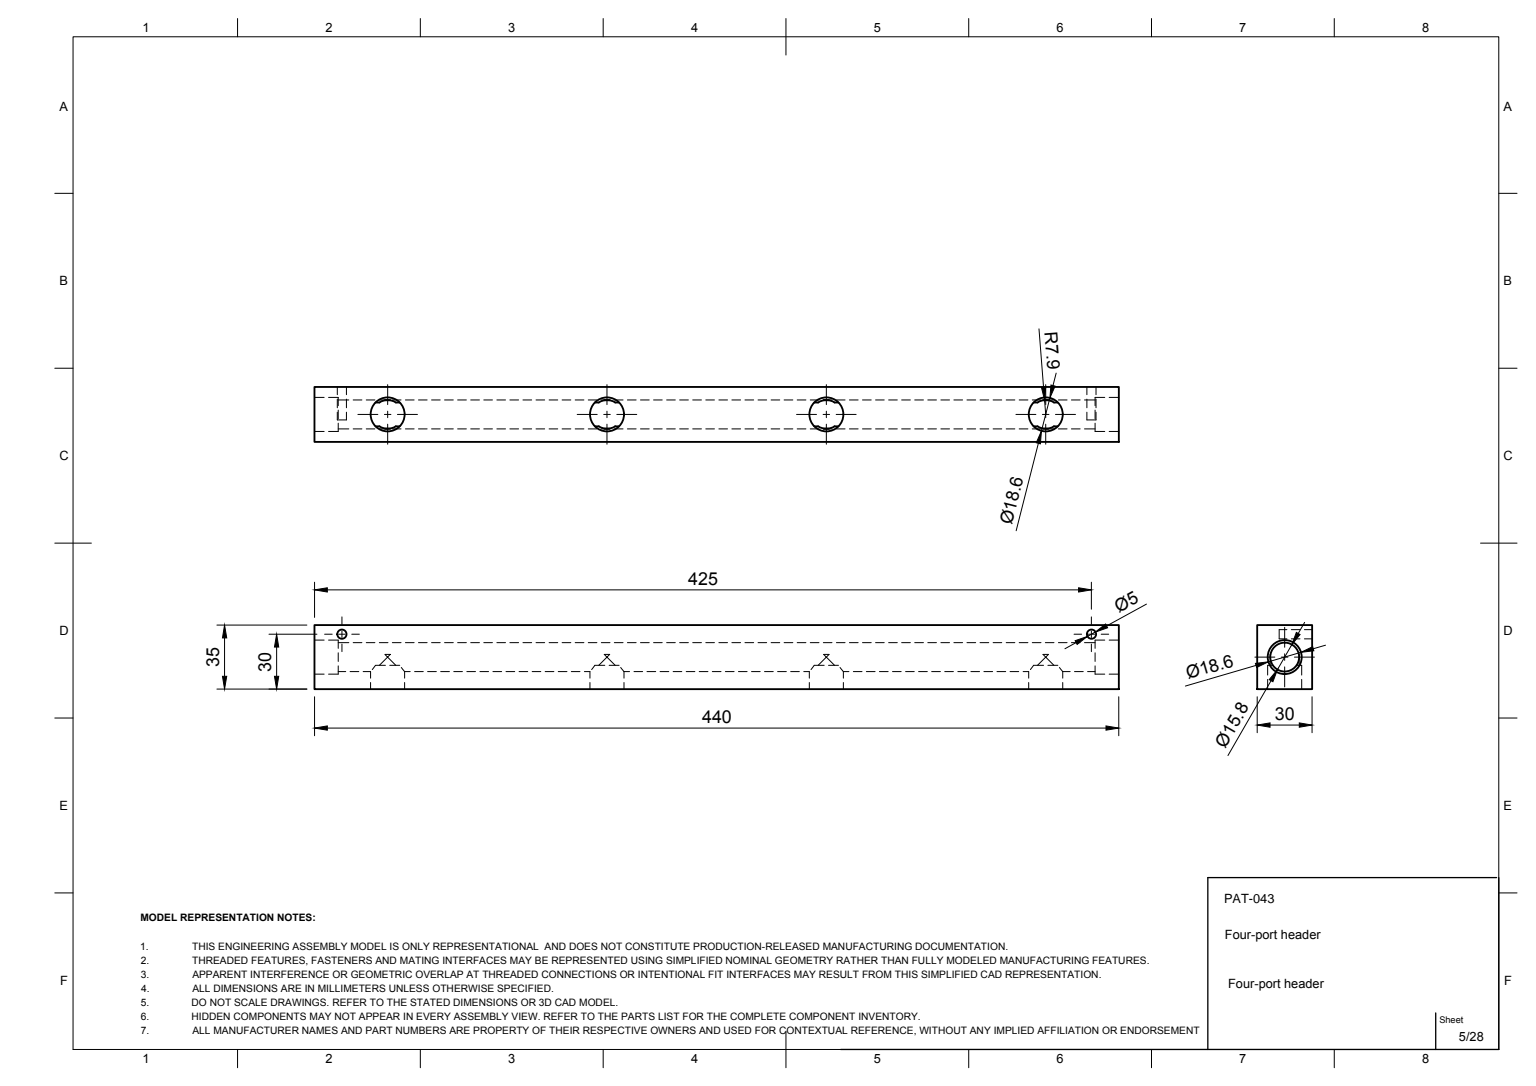
ISO-10303-21;
HEADER;
/* Generated by software containing ST-Developer
 * from STEP Tools, Inc. (www.steptools.com) 
 */

FILE_DESCRIPTION(
/* description */ ('Four-valve pipe header'),
/* implementation_level */ '2;1');

FILE_NAME(
/* name */ 'Four-port header.step',
/* time_stamp */ '2026-10-29T16:56:19-07:00',
/* author */ (''),
/* organization */ (''),
/* preprocessor_version */ 'ST-DEVELOPER v20.2',
/* originating_system */ 'Autodesk Translation Framework v15.17.0.0',
/* authorisation */ '');

FILE_SCHEMA (('AUTOMOTIVE_DESIGN { 1 0 10303 214 3 1 1 }'));
ENDSEC;

DATA;
#10=MECHANICAL_DESIGN_GEOMETRIC_PRESENTATION_REPRESENTATION('',(#333),#10119);
#281=SHAPE_REPRESENTATION_RELATIONSHIP('SRR','None',#10242,#307);
#307=ADVANCED_BREP_SHAPE_REPRESENTATION('',(#359),#10091);
#333=STYLED_ITEM('',(#10484),#359);
#359=MANIFOLD_SOLID_BREP('Body1',#5579);
#382=B_SPLINE_CURVE_WITH_KNOTS('',3,(#8408,#8409,#8410,#8411,#8412,#8413,
#8414,#8415),.UNSPECIFIED.,.F.,.F.,(4,2,2,4),(3.10041913490528,3.25801314591541,
3.57457123454079,3.89112932316618),.UNSPECIFIED.);
#383=B_SPLINE_CURVE_WITH_KNOTS('',3,(#8417,#8418,#8419,#8420,#8421,#8422,
#8423,#8424),.UNSPECIFIED.,.F.,.F.,(4,2,2,4),(3.89112932316618,4.20768741179156,
4.52424550041694,4.68183951142707),.UNSPECIFIED.);
#384=B_SPLINE_CURVE_WITH_KNOTS('',3,(#8439,#8440,#8441,#8442,#8443,#8444,
#8445,#8446,#8447,#8448,#8449,#8450,#8451,#8452),.UNSPECIFIED.,.F.,.F.,
(4,2,2,2,2,2,4),(0.506332919461168,0.663926930471297,0.980485019096678,
1.29704310772206,1.61360119634744,1.93015928497282,2.08775329598295),
 .UNSPECIFIED.);
#385=B_SPLINE_CURVE_WITH_KNOTS('',3,(#8463,#8464,#8465,#8466,#8467,#8468,
#8469,#8470),.UNSPECIFIED.,.F.,.F.,(4,2,2,4),(3.10041913490528,3.25801314591541,
3.5745712345408,3.89112932316618),.UNSPECIFIED.);
#386=B_SPLINE_CURVE_WITH_KNOTS('',3,(#8472,#8473,#8474,#8475,#8476,#8477,
#8478,#8479),.UNSPECIFIED.,.F.,.F.,(4,2,2,4),(3.89112932316618,4.20768741179156,
4.52424550041694,4.68183951142707),.UNSPECIFIED.);
#387=B_SPLINE_CURVE_WITH_KNOTS('',3,(#8494,#8495,#8496,#8497,#8498,#8499,
#8500,#8501,#8502,#8503,#8504,#8505,#8506,#8507),.UNSPECIFIED.,.F.,.F.,
(4,2,2,2,2,2,4),(0.506332919461167,0.663926930471296,0.980485019096678,
1.29704310772206,1.61360119634744,1.93015928497282,2.08775329598295),
 .UNSPECIFIED.);
#388=B_SPLINE_CURVE_WITH_KNOTS('',3,(#8518,#8519,#8520,#8521,#8522,#8523,
#8524,#8525),.UNSPECIFIED.,.F.,.F.,(4,2,2,4),(3.10041913490528,3.25801314591541,
3.5745712345408,3.89112932316618),.UNSPECIFIED.);
#389=B_SPLINE_CURVE_WITH_KNOTS('',3,(#8527,#8528,#8529,#8530,#8531,#8532,
#8533,#8534),.UNSPECIFIED.,.F.,.F.,(4,2,2,4),(3.89112932316618,4.20768741179156,
4.52424550041694,4.68183951142707),.UNSPECIFIED.);
#390=B_SPLINE_CURVE_WITH_KNOTS('',3,(#8549,#8550,#8551,#8552,#8553,#8554,
#8555,#8556,#8557,#8558,#8559,#8560,#8561,#8562),.UNSPECIFIED.,.F.,.F.,
(4,2,2,2,2,2,4),(0.506332919461169,0.663926930471296,0.980485019096678,
1.29704310772206,1.61360119634744,1.93015928497282,2.08775329598295),
 .UNSPECIFIED.);
#391=B_SPLINE_CURVE_WITH_KNOTS('',3,(#8570,#8571,#8572,#8573,#8574,#8575,
#8576,#8577),.UNSPECIFIED.,.F.,.F.,(4,2,2,4),(3.10041913490528,3.25801314591541,
3.5745712345408,3.89112932316618),.UNSPECIFIED.);
#392=B_SPLINE_CURVE_WITH_KNOTS('',3,(#8579,#8580,#8581,#8582,#8583,#8584,
#8585,#8586),.UNSPECIFIED.,.F.,.F.,(4,2,2,4),(3.89112932316618,4.20768741179156,
4.52424550041694,4.68183951142707),.UNSPECIFIED.);
#393=B_SPLINE_CURVE_WITH_KNOTS('',3,(#8591,#8592,#8593,#8594,#8595,#8596,
#8597,#8598,#8599,#8600,#8601,#8602,#8603,#8604),.UNSPECIFIED.,.F.,.F.,
(4,2,2,2,2,2,4),(0.506332919461165,0.663926930471296,0.980485019096678,
1.29704310772206,1.61360119634744,1.93015928497282,2.08775329598295),
 .UNSPECIFIED.);
#394=ELLIPSE('',#5919,1.11722871427474,0.789999999999999);
#395=ELLIPSE('',#5920,1.11722871427474,0.789999999999999);
#396=ELLIPSE('',#5922,1.11722871427474,0.789999999999999);
#397=ELLIPSE('',#5924,1.11722871427474,0.789999999999999);
#398=ELLIPSE('',#5926,1.11722871427474,0.789999999999999);
#399=ELLIPSE('',#5927,1.11722871427474,0.789999999999999);
#400=ELLIPSE('',#5930,1.11722871427474,0.789999999999999);
#401=ELLIPSE('',#5931,1.11722871427474,0.789999999999999);
#402=ELLIPSE('',#5935,1.11722871427474,0.79);
#403=ELLIPSE('',#5936,1.11722871427474,0.79);
#404=ELLIPSE('',#5937,1.11722871427475,0.79);
#405=ELLIPSE('',#5938,1.11722871427474,0.79);
#406=ELLIPSE('',#5939,1.11722871427475,0.79);
#407=ELLIPSE('',#5940,1.11722871427475,0.79);
#408=ELLIPSE('',#5941,1.11722871427474,0.789999999999999);
#409=ELLIPSE('',#5942,1.11722871427474,0.789999999999999);
#410=ELLIPSE('',#5943,1.11722871427474,0.789999999999999);
#411=ELLIPSE('',#5944,1.11722871427474,0.789999999999999);
#412=ELLIPSE('',#5945,1.11722871427474,0.789999999999999);
#413=ELLIPSE('',#5946,1.11722871427474,0.789999999999999);
#414=ELLIPSE('',#5947,1.11722871427474,0.789999999999999);
#415=ELLIPSE('',#5948,1.11722871427474,0.789999999999999);
#416=ELLIPSE('',#5949,1.11722871427474,0.789999999999999);
#417=ELLIPSE('',#5950,1.11722871427474,0.789999999999999);
#418=ELLIPSE('',#5951,1.11722871427474,0.789999999999999);
#419=ELLIPSE('',#5952,1.11722871427474,0.789999999999999);
#420=ELLIPSE('',#5953,1.11722871427474,0.789999999999999);
#421=ELLIPSE('',#5954,1.11722871427474,0.789999999999999);
#422=ELLIPSE('',#5955,1.11722871427474,0.789999999999999);
#423=ELLIPSE('',#5956,1.11722871427474,0.789999999999999);
#424=ELLIPSE('',#5957,1.11722871427474,0.79);
#425=ELLIPSE('',#5958,1.11722871427475,0.79);
#426=FACE_BOUND('',#1085,.T.);
#427=FACE_BOUND('',#1088,.T.);
#428=FACE_BOUND('',#1128,.T.);
#429=FACE_BOUND('',#1130,.T.);
#430=FACE_BOUND('',#1131,.T.);
#431=FACE_BOUND('',#1132,.T.);
#432=FACE_BOUND('',#1133,.T.);
#433=FACE_BOUND('',#1135,.T.);
#434=FACE_BOUND('',#1138,.T.);
#435=FACE_BOUND('',#1139,.T.);
#535=PLANE('',#5901);
#536=PLANE('',#5905);
#537=PLANE('',#5909);
#538=PLANE('',#5914);
#539=PLANE('',#5916);
#540=PLANE('',#5933);
#541=PLANE('',#5959);
#542=PLANE('',#5964);
#543=PLANE('',#5965);
#544=PLANE('',#5974);
#545=PLANE('',#5975);
#546=PLANE('',#5980);
#547=PLANE('',#5981);
#548=PLANE('',#5990);
#549=PLANE('',#5991);
#550=PLANE('',#5996);
#551=PLANE('',#5997);
#552=PLANE('',#6006);
#553=PLANE('',#6007);
#554=PLANE('',#6012);
#555=PLANE('',#6013);
#556=PLANE('',#6014);
#557=PLANE('',#6015);
#558=PLANE('',#6016);
#559=PLANE('',#6017);
#560=PLANE('',#6018);
#747=FACE_OUTER_BOUND('',#1079,.T.);
#748=FACE_OUTER_BOUND('',#1080,.T.);
#749=FACE_OUTER_BOUND('',#1081,.T.);
#750=FACE_OUTER_BOUND('',#1082,.T.);
#751=FACE_OUTER_BOUND('',#1083,.T.);
#752=FACE_OUTER_BOUND('',#1084,.T.);
#753=FACE_OUTER_BOUND('',#1086,.T.);
#754=FACE_OUTER_BOUND('',#1087,.T.);
#755=FACE_OUTER_BOUND('',#1089,.T.);
#756=FACE_OUTER_BOUND('',#1090,.T.);
#757=FACE_OUTER_BOUND('',#1091,.T.);
#758=FACE_OUTER_BOUND('',#1092,.T.);
#759=FACE_OUTER_BOUND('',#1093,.T.);
#760=FACE_OUTER_BOUND('',#1094,.T.);
#761=FACE_OUTER_BOUND('',#1095,.T.);
#762=FACE_OUTER_BOUND('',#1096,.T.);
#763=FACE_OUTER_BOUND('',#1097,.T.);
#764=FACE_OUTER_BOUND('',#1098,.T.);
#765=FACE_OUTER_BOUND('',#1099,.T.);
#766=FACE_OUTER_BOUND('',#1100,.T.);
#767=FACE_OUTER_BOUND('',#1101,.T.);
#768=FACE_OUTER_BOUND('',#1102,.T.);
#769=FACE_OUTER_BOUND('',#1103,.T.);
#770=FACE_OUTER_BOUND('',#1104,.T.);
#771=FACE_OUTER_BOUND('',#1105,.T.);
#772=FACE_OUTER_BOUND('',#1106,.T.);
#773=FACE_OUTER_BOUND('',#1107,.T.);
#774=FACE_OUTER_BOUND('',#1108,.T.);
#775=FACE_OUTER_BOUND('',#1109,.T.);
#776=FACE_OUTER_BOUND('',#1110,.T.);
#777=FACE_OUTER_BOUND('',#1111,.T.);
#778=FACE_OUTER_BOUND('',#1112,.T.);
#779=FACE_OUTER_BOUND('',#1113,.T.);
#780=FACE_OUTER_BOUND('',#1114,.T.);
#781=FACE_OUTER_BOUND('',#1115,.T.);
#782=FACE_OUTER_BOUND('',#1116,.T.);
#783=FACE_OUTER_BOUND('',#1117,.T.);
#784=FACE_OUTER_BOUND('',#1118,.T.);
#785=FACE_OUTER_BOUND('',#1119,.T.);
#786=FACE_OUTER_BOUND('',#1120,.T.);
#787=FACE_OUTER_BOUND('',#1121,.T.);
#788=FACE_OUTER_BOUND('',#1122,.T.);
#789=FACE_OUTER_BOUND('',#1123,.T.);
#790=FACE_OUTER_BOUND('',#1124,.T.);
#791=FACE_OUTER_BOUND('',#1125,.T.);
#792=FACE_OUTER_BOUND('',#1126,.T.);
#793=FACE_OUTER_BOUND('',#1127,.T.);
#794=FACE_OUTER_BOUND('',#1129,.T.);
#795=FACE_OUTER_BOUND('',#1134,.T.);
#796=FACE_OUTER_BOUND('',#1136,.T.);
#797=FACE_OUTER_BOUND('',#1137,.T.);
#1079=EDGE_LOOP('',(#3741,#3742,#3743,#3744));
#1080=EDGE_LOOP('',(#3745));
#1081=EDGE_LOOP('',(#3746,#3747,#3748,#3749));
#1082=EDGE_LOOP('',(#3750));
#1083=EDGE_LOOP('',(#3751,#3752,#3753,#3754));
#1084=EDGE_LOOP('',(#3755));
#1085=EDGE_LOOP('',(#3756));
#1086=EDGE_LOOP('',(#3757,#3758,#3759,#3760));
#1087=EDGE_LOOP('',(#3761));
#1088=EDGE_LOOP('',(#3762));
#1089=EDGE_LOOP('',(#3763,#3764));
#1090=EDGE_LOOP('',(#3765,#3766,#3767));
#1091=EDGE_LOOP('',(#3768,#3769,#3770));
#1092=EDGE_LOOP('',(#3771,#3772,#3773));
#1093=EDGE_LOOP('',(#3774,#3775,#3776));
#1094=EDGE_LOOP('',(#3777,#3778));
#1095=EDGE_LOOP('',(#3779,#3780,#3781,#3782,#3783,#3784,#3785,#3786,#3787,
#3788,#3789,#3790,#3791,#3792,#3793,#3794,#3795,#3796,#3797,#3798,#3799,
#3800,#3801,#3802,#3803,#3804,#3805,#3806,#3807,#3808,#3809,#3810,#3811,
#3812,#3813,#3814,#3815,#3816,#3817,#3818,#3819,#3820,#3821,#3822,#3823,
#3824,#3825,#3826,#3827,#3828,#3829,#3830,#3831,#3832,#3833,#3834,#3835,
#3836,#3837,#3838,#3839,#3840,#3841,#3842,#3843,#3844,#3845,#3846,#3847,
#3848,#3849,#3850,#3851,#3852,#3853,#3854,#3855,#3856,#3857,#3858));
#1096=EDGE_LOOP('',(#3859,#3860,#3861,#3862));
#1097=EDGE_LOOP('',(#3863,#3864,#3865,#3866,#3867,#3868,#3869,#3870));
#1098=EDGE_LOOP('',(#3871,#3872,#3873,#3874));
#1099=EDGE_LOOP('',(#3875,#3876));
#1100=EDGE_LOOP('',(#3877,#3878,#3879));
#1101=EDGE_LOOP('',(#3880,#3881,#3882));
#1102=EDGE_LOOP('',(#3883,#3884,#3885));
#1103=EDGE_LOOP('',(#3886,#3887,#3888));
#1104=EDGE_LOOP('',(#3889,#3890));
#1105=EDGE_LOOP('',(#3891,#3892,#3893,#3894));
#1106=EDGE_LOOP('',(#3895,#3896,#3897,#3898,#3899,#3900,#3901,#3902));
#1107=EDGE_LOOP('',(#3903,#3904,#3905,#3906));
#1108=EDGE_LOOP('',(#3907,#3908));
#1109=EDGE_LOOP('',(#3909,#3910,#3911));
#1110=EDGE_LOOP('',(#3912,#3913,#3914));
#1111=EDGE_LOOP('',(#3915,#3916,#3917));
#1112=EDGE_LOOP('',(#3918,#3919,#3920));
#1113=EDGE_LOOP('',(#3921,#3922));
#1114=EDGE_LOOP('',(#3923,#3924,#3925,#3926));
#1115=EDGE_LOOP('',(#3927,#3928,#3929,#3930,#3931,#3932,#3933,#3934));
#1116=EDGE_LOOP('',(#3935,#3936,#3937,#3938));
#1117=EDGE_LOOP('',(#3939,#3940));
#1118=EDGE_LOOP('',(#3941,#3942,#3943));
#1119=EDGE_LOOP('',(#3944,#3945,#3946));
#1120=EDGE_LOOP('',(#3947,#3948,#3949));
#1121=EDGE_LOOP('',(#3950,#3951,#3952));
#1122=EDGE_LOOP('',(#3953,#3954));
#1123=EDGE_LOOP('',(#3955,#3956,#3957,#3958));
#1124=EDGE_LOOP('',(#3959,#3960,#3961,#3962,#3963,#3964,#3965,#3966));
#1125=EDGE_LOOP('',(#3967,#3968,#3969,#3970));
#1126=EDGE_LOOP('',(#3971,#3972,#3973,#3974));
#1127=EDGE_LOOP('',(#3975,#3976,#3977,#3978));
#1128=EDGE_LOOP('',(#3979));
#1129=EDGE_LOOP('',(#3980,#3981,#3982,#3983));
#1130=EDGE_LOOP('',(#3984));
#1131=EDGE_LOOP('',(#3985));
#1132=EDGE_LOOP('',(#3986));
#1133=EDGE_LOOP('',(#3987));
#1134=EDGE_LOOP('',(#3988,#3989,#3990,#3991));
#1135=EDGE_LOOP('',(#3992));
#1136=EDGE_LOOP('',(#3993,#3994,#3995,#3996));
#1137=EDGE_LOOP('',(#3997,#3998,#3999,#4000));
#1138=EDGE_LOOP('',(#4001));
#1139=EDGE_LOOP('',(#4002));
#1520=LINE('',#8342,#1938);
#1521=LINE('',#8349,#1939);
#1522=LINE('',#8356,#1940);
#1523=LINE('',#8365,#1941);
#1524=LINE('',#8373,#1942);
#1525=LINE('',#8399,#1943);
#1526=LINE('',#8402,#1944);
#1527=LINE('',#8406,#1945);
#1528=LINE('',#8426,#1946);
#1529=LINE('',#8432,#1947);
#1530=LINE('',#8437,#1948);
#1531=LINE('',#8454,#1949);
#1532=LINE('',#8457,#1950);
#1533=LINE('',#8461,#1951);
#1534=LINE('',#8481,#1952);
#1535=LINE('',#8487,#1953);
#1536=LINE('',#8492,#1954);
#1537=LINE('',#8509,#1955);
#1538=LINE('',#8512,#1956);
#1539=LINE('',#8516,#1957);
#1540=LINE('',#8536,#1958);
#1541=LINE('',#8542,#1959);
#1542=LINE('',#8547,#1960);
#1543=LINE('',#8564,#1961);
#1544=LINE('',#8566,#1962);
#1545=LINE('',#8568,#1963);
#1546=LINE('',#8587,#1964);
#1547=LINE('',#8589,#1965);
#1548=LINE('',#8605,#1966);
#1549=LINE('',#8606,#1967);
#1550=LINE('',#8610,#1968);
#1551=LINE('',#8615,#1969);
#1552=LINE('',#8620,#1970);
#1553=LINE('',#8627,#1971);
#1554=LINE('',#8645,#1972);
#1555=LINE('',#8663,#1973);
#1556=LINE('',#8681,#1974);
#1557=LINE('',#8687,#1975);
#1558=LINE('',#8689,#1976);
#1559=LINE('',#8691,#1977);
#1560=LINE('',#8692,#1978);
#1561=LINE('',#8695,#1979);
#1562=LINE('',#8697,#1980);
#1563=LINE('',#8698,#1981);
#1564=LINE('',#8701,#1982);
#1565=LINE('',#8703,#1983);
#1566=LINE('',#8704,#1984);
#1567=LINE('',#8706,#1985);
#1568=LINE('',#8707,#1986);
#1938=VECTOR('',#6579,0.25);
#1939=VECTOR('',#6588,0.25);
#1940=VECTOR('',#6597,0.93);
#1941=VECTOR('',#6608,0.93);
#1942=VECTOR('',#6617,1.);
#1943=VECTOR('',#6652,1.);
#1944=VECTOR('',#6655,0.79);
#1945=VECTOR('',#6658,1.);
#1946=VECTOR('',#6659,1.);
#1947=VECTOR('',#6664,1.);
#1948=VECTOR('',#6669,1.);
#1949=VECTOR('',#6670,1.);
#1950=VECTOR('',#6673,0.79);
#1951=VECTOR('',#6676,1.);
#1952=VECTOR('',#6677,1.);
#1953=VECTOR('',#6682,1.);
#1954=VECTOR('',#6687,1.);
#1955=VECTOR('',#6688,1.);
#1956=VECTOR('',#6691,0.79);
#1957=VECTOR('',#6694,1.);
#1958=VECTOR('',#6695,1.);
#1959=VECTOR('',#6700,1.);
#1960=VECTOR('',#6705,1.);
#1961=VECTOR('',#6706,1.);
#1962=VECTOR('',#6709,0.79);
#1963=VECTOR('',#6710,1.);
#1964=VECTOR('',#6711,1.);
#1965=VECTOR('',#6712,1.);
#1966=VECTOR('',#6713,1.);
#1967=VECTOR('',#6714,0.79);
#1968=VECTOR('',#6717,1.);
#1969=VECTOR('',#6722,1.);
#1970=VECTOR('',#6727,1.);
#1971=VECTOR('',#6738,0.93);
#1972=VECTOR('',#6771,0.93);
#1973=VECTOR('',#6804,0.93);
#1974=VECTOR('',#6837,0.93);
#1975=VECTOR('',#6844,1.);
#1976=VECTOR('',#6845,1.);
#1977=VECTOR('',#6846,1.);
#1978=VECTOR('',#6847,1.);
#1979=VECTOR('',#6850,1.);
#1980=VECTOR('',#6851,1.);
#1981=VECTOR('',#6852,1.);
#1982=VECTOR('',#6855,1.);
#1983=VECTOR('',#6856,1.);
#1984=VECTOR('',#6857,1.);
#1985=VECTOR('',#6860,1.);
#1986=VECTOR('',#6861,1.);
#2356=CIRCLE('',#5899,0.25);
#2357=CIRCLE('',#5900,0.25);
#2358=CIRCLE('',#5903,0.25);
#2359=CIRCLE('',#5904,0.25);
#2360=CIRCLE('',#5907,0.93);
#2361=CIRCLE('',#5908,0.93);
#2362=CIRCLE('',#5910,0.79);
#2363=CIRCLE('',#5912,0.93);
#2364=CIRCLE('',#5913,0.93);
#2365=CIRCLE('',#5915,0.79);
#2366=CIRCLE('',#5917,0.789999999999999);
#2367=CIRCLE('',#5923,0.789999999999999);
#2368=CIRCLE('',#5928,0.789999999999999);
#2369=CIRCLE('',#5932,0.789999999999999);
#2370=CIRCLE('',#5960,0.93);
#2371=CIRCLE('',#5962,0.93);
#2372=CIRCLE('',#5963,0.93);
#2373=CIRCLE('',#5966,0.789999999999999);
#2374=CIRCLE('',#5969,0.789999999999999);
#2375=CIRCLE('',#5971,0.789999999999999);
#2376=CIRCLE('',#5973,0.789999999999999);
#2377=CIRCLE('',#5976,0.93);
#2378=CIRCLE('',#5978,0.93);
#2379=CIRCLE('',#5979,0.93);
#2380=CIRCLE('',#5982,0.789999999999999);
#2381=CIRCLE('',#5985,0.789999999999999);
#2382=CIRCLE('',#5987,0.789999999999999);
#2383=CIRCLE('',#5989,0.789999999999999);
#2384=CIRCLE('',#5992,0.93);
#2385=CIRCLE('',#5994,0.93);
#2386=CIRCLE('',#5995,0.93);
#2387=CIRCLE('',#5998,0.79);
#2388=CIRCLE('',#6001,0.79);
#2389=CIRCLE('',#6003,0.79);
#2390=CIRCLE('',#6005,0.79);
#2391=CIRCLE('',#6008,0.93);
#2392=CIRCLE('',#6010,0.93);
#2393=CIRCLE('',#6011,0.93);
#2580=VERTEX_POINT('',#8339);
#2581=VERTEX_POINT('',#8341);
#2582=VERTEX_POINT('',#8346);
#2583=VERTEX_POINT('',#8348);
#2584=VERTEX_POINT('',#8353);
#2585=VERTEX_POINT('',#8355);
#2586=VERTEX_POINT('',#8359);
#2587=VERTEX_POINT('',#8362);
#2588=VERTEX_POINT('',#8364);
#2589=VERTEX_POINT('',#8368);
#2590=VERTEX_POINT('',#8371);
#2591=VERTEX_POINT('',#8372);
#2592=VERTEX_POINT('',#8376);
#2593=VERTEX_POINT('',#8380);
#2594=VERTEX_POINT('',#8381);
#2595=VERTEX_POINT('',#8383);
#2596=VERTEX_POINT('',#8387);
#2597=VERTEX_POINT('',#8389);
#2598=VERTEX_POINT('',#8393);
#2599=VERTEX_POINT('',#8395);
#2600=VERTEX_POINT('',#8401);
#2601=VERTEX_POINT('',#8403);
#2602=VERTEX_POINT('',#8405);
#2603=VERTEX_POINT('',#8407);
#2604=VERTEX_POINT('',#8416);
#2605=VERTEX_POINT('',#8425);
#2606=VERTEX_POINT('',#8427);
#2607=VERTEX_POINT('',#8429);
#2608=VERTEX_POINT('',#8431);
#2609=VERTEX_POINT('',#8434);
#2610=VERTEX_POINT('',#8436);
#2611=VERTEX_POINT('',#8438);
#2612=VERTEX_POINT('',#8453);
#2613=VERTEX_POINT('',#8456);
#2614=VERTEX_POINT('',#8458);
#2615=VERTEX_POINT('',#8460);
#2616=VERTEX_POINT('',#8462);
#2617=VERTEX_POINT('',#8471);
#2618=VERTEX_POINT('',#8480);
#2619=VERTEX_POINT('',#8482);
#2620=VERTEX_POINT('',#8484);
#2621=VERTEX_POINT('',#8486);
#2622=VERTEX_POINT('',#8489);
#2623=VERTEX_POINT('',#8491);
#2624=VERTEX_POINT('',#8493);
#2625=VERTEX_POINT('',#8508);
#2626=VERTEX_POINT('',#8511);
#2627=VERTEX_POINT('',#8513);
#2628=VERTEX_POINT('',#8515);
#2629=VERTEX_POINT('',#8517);
#2630=VERTEX_POINT('',#8526);
#2631=VERTEX_POINT('',#8535);
#2632=VERTEX_POINT('',#8537);
#2633=VERTEX_POINT('',#8539);
#2634=VERTEX_POINT('',#8541);
#2635=VERTEX_POINT('',#8544);
#2636=VERTEX_POINT('',#8546);
#2637=VERTEX_POINT('',#8548);
#2638=VERTEX_POINT('',#8563);
#2639=VERTEX_POINT('',#8567);
#2640=VERTEX_POINT('',#8569);
#2641=VERTEX_POINT('',#8578);
#2642=VERTEX_POINT('',#8588);
#2643=VERTEX_POINT('',#8590);
#2644=VERTEX_POINT('',#8607);
#2645=VERTEX_POINT('',#8609);
#2646=VERTEX_POINT('',#8612);
#2647=VERTEX_POINT('',#8614);
#2648=VERTEX_POINT('',#8617);
#2649=VERTEX_POINT('',#8619);
#2650=VERTEX_POINT('',#8625);
#2651=VERTEX_POINT('',#8643);
#2652=VERTEX_POINT('',#8661);
#2653=VERTEX_POINT('',#8679);
#2654=VERTEX_POINT('',#8685);
#2655=VERTEX_POINT('',#8686);
#2656=VERTEX_POINT('',#8688);
#2657=VERTEX_POINT('',#8690);
#2658=VERTEX_POINT('',#8694);
#2659=VERTEX_POINT('',#8696);
#2660=VERTEX_POINT('',#8700);
#2661=VERTEX_POINT('',#8702);
#3037=EDGE_CURVE('',#2580,#2580,#2356,.T.);
#3038=EDGE_CURVE('',#2580,#2581,#1520,.T.);
#3039=EDGE_CURVE('',#2581,#2581,#2357,.T.);
#3040=EDGE_CURVE('',#2582,#2582,#2358,.T.);
#3041=EDGE_CURVE('',#2582,#2583,#1521,.T.);
#3042=EDGE_CURVE('',#2583,#2583,#2359,.T.);
#3043=EDGE_CURVE('',#2584,#2584,#2360,.T.);
#3044=EDGE_CURVE('',#2584,#2585,#1522,.T.);
#3045=EDGE_CURVE('',#2585,#2585,#2361,.T.);
#3046=EDGE_CURVE('',#2586,#2586,#2362,.T.);
#3047=EDGE_CURVE('',#2587,#2587,#2363,.T.);
#3048=EDGE_CURVE('',#2587,#2588,#1523,.T.);
#3049=EDGE_CURVE('',#2588,#2588,#2364,.T.);
#3050=EDGE_CURVE('',#2589,#2589,#2365,.T.);
#3051=EDGE_CURVE('',#2590,#2591,#1524,.T.);
#3052=EDGE_CURVE('',#2591,#2590,#2366,.T.);
#3053=EDGE_CURVE('',#2591,#2592,#394,.T.);
#3054=EDGE_CURVE('',#2592,#2590,#395,.T.);
#3055=EDGE_CURVE('',#2593,#2594,#396,.T.);
#3056=EDGE_CURVE('',#2593,#2595,#2367,.T.);
#3057=EDGE_CURVE('',#2594,#2595,#397,.T.);
#3058=EDGE_CURVE('',#2592,#2596,#398,.T.);
#3059=EDGE_CURVE('',#2597,#2592,#399,.T.);
#3060=EDGE_CURVE('',#2596,#2597,#2368,.T.);
#3061=EDGE_CURVE('',#2594,#2598,#400,.T.);
#3062=EDGE_CURVE('',#2599,#2594,#401,.T.);
#3063=EDGE_CURVE('',#2598,#2599,#2369,.T.);
#3064=EDGE_CURVE('',#2595,#2593,#1525,.T.);
#3065=EDGE_CURVE('',#2589,#2600,#1526,.T.);
#3066=EDGE_CURVE('',#2600,#2601,#402,.T.);
#3067=EDGE_CURVE('',#2601,#2602,#1527,.T.);
#3068=EDGE_CURVE('',#2602,#2603,#382,.T.);
#3069=EDGE_CURVE('',#2603,#2604,#383,.T.);
#3070=EDGE_CURVE('',#2604,#2605,#1528,.T.);
#3071=EDGE_CURVE('',#2605,#2606,#403,.T.);
#3072=EDGE_CURVE('',#2606,#2607,#404,.T.);
#3073=EDGE_CURVE('',#2607,#2608,#1529,.T.);
#3074=EDGE_CURVE('',#2608,#2606,#405,.T.);
#3075=EDGE_CURVE('',#2606,#2609,#406,.T.);
#3076=EDGE_CURVE('',#2609,#2610,#1530,.T.);
#3077=EDGE_CURVE('',#2610,#2611,#384,.T.);
#3078=EDGE_CURVE('',#2611,#2612,#1531,.T.);
#3079=EDGE_CURVE('',#2612,#2600,#407,.T.);
#3080=EDGE_CURVE('',#2600,#2613,#1532,.T.);
#3081=EDGE_CURVE('',#2613,#2614,#408,.T.);
#3082=EDGE_CURVE('',#2614,#2615,#1533,.T.);
#3083=EDGE_CURVE('',#2615,#2616,#385,.T.);
#3084=EDGE_CURVE('',#2616,#2617,#386,.T.);
#3085=EDGE_CURVE('',#2617,#2618,#1534,.T.);
#3086=EDGE_CURVE('',#2618,#2619,#409,.T.);
#3087=EDGE_CURVE('',#2619,#2620,#410,.T.);
#3088=EDGE_CURVE('',#2620,#2621,#1535,.T.);
#3089=EDGE_CURVE('',#2621,#2619,#411,.T.);
#3090=EDGE_CURVE('',#2619,#2622,#412,.T.);
#3091=EDGE_CURVE('',#2622,#2623,#1536,.T.);
#3092=EDGE_CURVE('',#2623,#2624,#387,.T.);
#3093=EDGE_CURVE('',#2624,#2625,#1537,.T.);
#3094=EDGE_CURVE('',#2625,#2613,#413,.T.);
#3095=EDGE_CURVE('',#2613,#2626,#1538,.T.);
#3096=EDGE_CURVE('',#2626,#2627,#414,.T.);
#3097=EDGE_CURVE('',#2627,#2628,#1539,.T.);
#3098=EDGE_CURVE('',#2628,#2629,#388,.T.);
#3099=EDGE_CURVE('',#2629,#2630,#389,.T.);
#3100=EDGE_CURVE('',#2630,#2631,#1540,.T.);
#3101=EDGE_CURVE('',#2631,#2632,#415,.T.);
#3102=EDGE_CURVE('',#2632,#2633,#416,.T.);
#3103=EDGE_CURVE('',#2633,#2634,#1541,.T.);
#3104=EDGE_CURVE('',#2634,#2632,#417,.T.);
#3105=EDGE_CURVE('',#2632,#2635,#418,.T.);
#3106=EDGE_CURVE('',#2635,#2636,#1542,.T.);
#3107=EDGE_CURVE('',#2636,#2637,#390,.T.);
#3108=EDGE_CURVE('',#2637,#2638,#1543,.T.);
#3109=EDGE_CURVE('',#2638,#2626,#419,.T.);
#3110=EDGE_CURVE('',#2626,#2594,#1544,.T.);
#3111=EDGE_CURVE('',#2598,#2639,#1545,.T.);
#3112=EDGE_CURVE('',#2639,#2640,#391,.T.);
#3113=EDGE_CURVE('',#2640,#2641,#392,.T.);
#3114=EDGE_CURVE('',#2641,#2597,#1546,.T.);
#3115=EDGE_CURVE('',#2596,#2642,#1547,.T.);
#3116=EDGE_CURVE('',#2642,#2643,#393,.T.);
#3117=EDGE_CURVE('',#2643,#2599,#1548,.T.);
#3118=EDGE_CURVE('',#2594,#2586,#1549,.T.);
#3119=EDGE_CURVE('',#2626,#2644,#420,.T.);
#3120=EDGE_CURVE('',#2644,#2645,#1550,.T.);
#3121=EDGE_CURVE('',#2645,#2626,#421,.T.);
#3122=EDGE_CURVE('',#2613,#2646,#422,.T.);
#3123=EDGE_CURVE('',#2646,#2647,#1551,.T.);
#3124=EDGE_CURVE('',#2647,#2613,#423,.T.);
#3125=EDGE_CURVE('',#2600,#2648,#424,.T.);
#3126=EDGE_CURVE('',#2648,#2649,#1552,.T.);
#3127=EDGE_CURVE('',#2649,#2600,#425,.T.);
#3128=EDGE_CURVE('',#2639,#2643,#2370,.T.);
#3129=EDGE_CURVE('',#2650,#2650,#2371,.T.);
#3130=EDGE_CURVE('',#2650,#2640,#1553,.T.);
#3131=EDGE_CURVE('',#2642,#2641,#2372,.T.);
#3132=EDGE_CURVE('',#2634,#2633,#2373,.T.);
#3133=EDGE_CURVE('',#2645,#2644,#2374,.T.);
#3134=EDGE_CURVE('',#2635,#2631,#2375,.T.);
#3135=EDGE_CURVE('',#2627,#2638,#2376,.T.);
#3136=EDGE_CURVE('',#2628,#2637,#2377,.T.);
#3137=EDGE_CURVE('',#2651,#2651,#2378,.T.);
#3138=EDGE_CURVE('',#2651,#2629,#1554,.T.);
#3139=EDGE_CURVE('',#2636,#2630,#2379,.T.);
#3140=EDGE_CURVE('',#2621,#2620,#2380,.T.);
#3141=EDGE_CURVE('',#2647,#2646,#2381,.T.);
#3142=EDGE_CURVE('',#2622,#2618,#2382,.T.);
#3143=EDGE_CURVE('',#2614,#2625,#2383,.T.);
#3144=EDGE_CURVE('',#2615,#2624,#2384,.T.);
#3145=EDGE_CURVE('',#2652,#2652,#2385,.T.);
#3146=EDGE_CURVE('',#2652,#2616,#1555,.T.);
#3147=EDGE_CURVE('',#2623,#2617,#2386,.T.);
#3148=EDGE_CURVE('',#2608,#2607,#2387,.T.);
#3149=EDGE_CURVE('',#2649,#2648,#2388,.T.);
#3150=EDGE_CURVE('',#2609,#2605,#2389,.T.);
#3151=EDGE_CURVE('',#2601,#2612,#2390,.T.);
#3152=EDGE_CURVE('',#2602,#2611,#2391,.T.);
#3153=EDGE_CURVE('',#2653,#2653,#2392,.T.);
#3154=EDGE_CURVE('',#2653,#2603,#1556,.T.);
#3155=EDGE_CURVE('',#2610,#2604,#2393,.T.);
#3156=EDGE_CURVE('',#2654,#2655,#1557,.T.);
#3157=EDGE_CURVE('',#2655,#2656,#1558,.T.);
#3158=EDGE_CURVE('',#2657,#2656,#1559,.T.);
#3159=EDGE_CURVE('',#2654,#2657,#1560,.T.);
#3160=EDGE_CURVE('',#2658,#2654,#1561,.T.);
#3161=EDGE_CURVE('',#2659,#2657,#1562,.T.);
#3162=EDGE_CURVE('',#2658,#2659,#1563,.T.);
#3163=EDGE_CURVE('',#2660,#2658,#1564,.T.);
#3164=EDGE_CURVE('',#2661,#2659,#1565,.T.);
#3165=EDGE_CURVE('',#2660,#2661,#1566,.T.);
#3166=EDGE_CURVE('',#2655,#2660,#1567,.T.);
#3167=EDGE_CURVE('',#2656,#2661,#1568,.T.);
#3741=ORIENTED_EDGE('',*,*,#3037,.F.);
#3742=ORIENTED_EDGE('',*,*,#3038,.T.);
#3743=ORIENTED_EDGE('',*,*,#3039,.T.);
#3744=ORIENTED_EDGE('',*,*,#3038,.F.);
#3745=ORIENTED_EDGE('',*,*,#3039,.F.);
#3746=ORIENTED_EDGE('',*,*,#3040,.F.);
#3747=ORIENTED_EDGE('',*,*,#3041,.T.);
#3748=ORIENTED_EDGE('',*,*,#3042,.T.);
#3749=ORIENTED_EDGE('',*,*,#3041,.F.);
#3750=ORIENTED_EDGE('',*,*,#3042,.F.);
#3751=ORIENTED_EDGE('',*,*,#3043,.F.);
#3752=ORIENTED_EDGE('',*,*,#3044,.T.);
#3753=ORIENTED_EDGE('',*,*,#3045,.F.);
#3754=ORIENTED_EDGE('',*,*,#3044,.F.);
#3755=ORIENTED_EDGE('',*,*,#3043,.T.);
#3756=ORIENTED_EDGE('',*,*,#3046,.F.);
#3757=ORIENTED_EDGE('',*,*,#3047,.F.);
#3758=ORIENTED_EDGE('',*,*,#3048,.T.);
#3759=ORIENTED_EDGE('',*,*,#3049,.T.);
#3760=ORIENTED_EDGE('',*,*,#3048,.F.);
#3761=ORIENTED_EDGE('',*,*,#3049,.F.);
#3762=ORIENTED_EDGE('',*,*,#3050,.F.);
#3763=ORIENTED_EDGE('',*,*,#3051,.F.);
#3764=ORIENTED_EDGE('',*,*,#3052,.F.);
#3765=ORIENTED_EDGE('',*,*,#3053,.F.);
#3766=ORIENTED_EDGE('',*,*,#3052,.T.);
#3767=ORIENTED_EDGE('',*,*,#3054,.F.);
#3768=ORIENTED_EDGE('',*,*,#3055,.F.);
#3769=ORIENTED_EDGE('',*,*,#3056,.T.);
#3770=ORIENTED_EDGE('',*,*,#3057,.F.);
#3771=ORIENTED_EDGE('',*,*,#3058,.F.);
#3772=ORIENTED_EDGE('',*,*,#3059,.F.);
#3773=ORIENTED_EDGE('',*,*,#3060,.F.);
#3774=ORIENTED_EDGE('',*,*,#3061,.F.);
#3775=ORIENTED_EDGE('',*,*,#3062,.F.);
#3776=ORIENTED_EDGE('',*,*,#3063,.F.);
#3777=ORIENTED_EDGE('',*,*,#3064,.F.);
#3778=ORIENTED_EDGE('',*,*,#3056,.F.);
#3779=ORIENTED_EDGE('',*,*,#3050,.T.);
#3780=ORIENTED_EDGE('',*,*,#3065,.T.);
#3781=ORIENTED_EDGE('',*,*,#3066,.T.);
#3782=ORIENTED_EDGE('',*,*,#3067,.T.);
#3783=ORIENTED_EDGE('',*,*,#3068,.T.);
#3784=ORIENTED_EDGE('',*,*,#3069,.T.);
#3785=ORIENTED_EDGE('',*,*,#3070,.T.);
#3786=ORIENTED_EDGE('',*,*,#3071,.T.);
#3787=ORIENTED_EDGE('',*,*,#3072,.T.);
#3788=ORIENTED_EDGE('',*,*,#3073,.T.);
#3789=ORIENTED_EDGE('',*,*,#3074,.T.);
#3790=ORIENTED_EDGE('',*,*,#3075,.T.);
#3791=ORIENTED_EDGE('',*,*,#3076,.T.);
#3792=ORIENTED_EDGE('',*,*,#3077,.T.);
#3793=ORIENTED_EDGE('',*,*,#3078,.T.);
#3794=ORIENTED_EDGE('',*,*,#3079,.T.);
#3795=ORIENTED_EDGE('',*,*,#3080,.T.);
#3796=ORIENTED_EDGE('',*,*,#3081,.T.);
#3797=ORIENTED_EDGE('',*,*,#3082,.T.);
#3798=ORIENTED_EDGE('',*,*,#3083,.T.);
#3799=ORIENTED_EDGE('',*,*,#3084,.T.);
#3800=ORIENTED_EDGE('',*,*,#3085,.T.);
#3801=ORIENTED_EDGE('',*,*,#3086,.T.);
#3802=ORIENTED_EDGE('',*,*,#3087,.T.);
#3803=ORIENTED_EDGE('',*,*,#3088,.T.);
#3804=ORIENTED_EDGE('',*,*,#3089,.T.);
#3805=ORIENTED_EDGE('',*,*,#3090,.T.);
#3806=ORIENTED_EDGE('',*,*,#3091,.T.);
#3807=ORIENTED_EDGE('',*,*,#3092,.T.);
#3808=ORIENTED_EDGE('',*,*,#3093,.T.);
#3809=ORIENTED_EDGE('',*,*,#3094,.T.);
#3810=ORIENTED_EDGE('',*,*,#3095,.T.);
#3811=ORIENTED_EDGE('',*,*,#3096,.T.);
#3812=ORIENTED_EDGE('',*,*,#3097,.T.);
#3813=ORIENTED_EDGE('',*,*,#3098,.T.);
#3814=ORIENTED_EDGE('',*,*,#3099,.T.);
#3815=ORIENTED_EDGE('',*,*,#3100,.T.);
#3816=ORIENTED_EDGE('',*,*,#3101,.T.);
#3817=ORIENTED_EDGE('',*,*,#3102,.T.);
#3818=ORIENTED_EDGE('',*,*,#3103,.T.);
#3819=ORIENTED_EDGE('',*,*,#3104,.T.);
#3820=ORIENTED_EDGE('',*,*,#3105,.T.);
#3821=ORIENTED_EDGE('',*,*,#3106,.T.);
#3822=ORIENTED_EDGE('',*,*,#3107,.T.);
#3823=ORIENTED_EDGE('',*,*,#3108,.T.);
#3824=ORIENTED_EDGE('',*,*,#3109,.T.);
#3825=ORIENTED_EDGE('',*,*,#3110,.T.);
#3826=ORIENTED_EDGE('',*,*,#3061,.T.);
#3827=ORIENTED_EDGE('',*,*,#3111,.T.);
#3828=ORIENTED_EDGE('',*,*,#3112,.T.);
#3829=ORIENTED_EDGE('',*,*,#3113,.T.);
#3830=ORIENTED_EDGE('',*,*,#3114,.T.);
#3831=ORIENTED_EDGE('',*,*,#3059,.T.);
#3832=ORIENTED_EDGE('',*,*,#3054,.T.);
#3833=ORIENTED_EDGE('',*,*,#3051,.T.);
#3834=ORIENTED_EDGE('',*,*,#3053,.T.);
#3835=ORIENTED_EDGE('',*,*,#3058,.T.);
#3836=ORIENTED_EDGE('',*,*,#3115,.T.);
#3837=ORIENTED_EDGE('',*,*,#3116,.T.);
#3838=ORIENTED_EDGE('',*,*,#3117,.T.);
#3839=ORIENTED_EDGE('',*,*,#3062,.T.);
#3840=ORIENTED_EDGE('',*,*,#3118,.T.);
#3841=ORIENTED_EDGE('',*,*,#3046,.T.);
#3842=ORIENTED_EDGE('',*,*,#3118,.F.);
#3843=ORIENTED_EDGE('',*,*,#3057,.T.);
#3844=ORIENTED_EDGE('',*,*,#3064,.T.);
#3845=ORIENTED_EDGE('',*,*,#3055,.T.);
#3846=ORIENTED_EDGE('',*,*,#3110,.F.);
#3847=ORIENTED_EDGE('',*,*,#3119,.T.);
#3848=ORIENTED_EDGE('',*,*,#3120,.T.);
#3849=ORIENTED_EDGE('',*,*,#3121,.T.);
#3850=ORIENTED_EDGE('',*,*,#3095,.F.);
#3851=ORIENTED_EDGE('',*,*,#3122,.T.);
#3852=ORIENTED_EDGE('',*,*,#3123,.T.);
#3853=ORIENTED_EDGE('',*,*,#3124,.T.);
#3854=ORIENTED_EDGE('',*,*,#3080,.F.);
#3855=ORIENTED_EDGE('',*,*,#3125,.T.);
#3856=ORIENTED_EDGE('',*,*,#3126,.T.);
#3857=ORIENTED_EDGE('',*,*,#3127,.T.);
#3858=ORIENTED_EDGE('',*,*,#3065,.F.);
#3859=ORIENTED_EDGE('',*,*,#3063,.T.);
#3860=ORIENTED_EDGE('',*,*,#3117,.F.);
#3861=ORIENTED_EDGE('',*,*,#3128,.F.);
#3862=ORIENTED_EDGE('',*,*,#3111,.F.);
#3863=ORIENTED_EDGE('',*,*,#3129,.F.);
#3864=ORIENTED_EDGE('',*,*,#3130,.T.);
#3865=ORIENTED_EDGE('',*,*,#3112,.F.);
#3866=ORIENTED_EDGE('',*,*,#3128,.T.);
#3867=ORIENTED_EDGE('',*,*,#3116,.F.);
#3868=ORIENTED_EDGE('',*,*,#3131,.T.);
#3869=ORIENTED_EDGE('',*,*,#3113,.F.);
#3870=ORIENTED_EDGE('',*,*,#3130,.F.);
#3871=ORIENTED_EDGE('',*,*,#3060,.T.);
#3872=ORIENTED_EDGE('',*,*,#3114,.F.);
#3873=ORIENTED_EDGE('',*,*,#3131,.F.);
#3874=ORIENTED_EDGE('',*,*,#3115,.F.);
#3875=ORIENTED_EDGE('',*,*,#3103,.F.);
#3876=ORIENTED_EDGE('',*,*,#3132,.F.);
#3877=ORIENTED_EDGE('',*,*,#3104,.F.);
#3878=ORIENTED_EDGE('',*,*,#3132,.T.);
#3879=ORIENTED_EDGE('',*,*,#3102,.F.);
#3880=ORIENTED_EDGE('',*,*,#3121,.F.);
#3881=ORIENTED_EDGE('',*,*,#3133,.T.);
#3882=ORIENTED_EDGE('',*,*,#3119,.F.);
#3883=ORIENTED_EDGE('',*,*,#3105,.F.);
#3884=ORIENTED_EDGE('',*,*,#3101,.F.);
#3885=ORIENTED_EDGE('',*,*,#3134,.F.);
#3886=ORIENTED_EDGE('',*,*,#3096,.F.);
#3887=ORIENTED_EDGE('',*,*,#3109,.F.);
#3888=ORIENTED_EDGE('',*,*,#3135,.F.);
#3889=ORIENTED_EDGE('',*,*,#3120,.F.);
#3890=ORIENTED_EDGE('',*,*,#3133,.F.);
#3891=ORIENTED_EDGE('',*,*,#3135,.T.);
#3892=ORIENTED_EDGE('',*,*,#3108,.F.);
#3893=ORIENTED_EDGE('',*,*,#3136,.F.);
#3894=ORIENTED_EDGE('',*,*,#3097,.F.);
#3895=ORIENTED_EDGE('',*,*,#3137,.F.);
#3896=ORIENTED_EDGE('',*,*,#3138,.T.);
#3897=ORIENTED_EDGE('',*,*,#3098,.F.);
#3898=ORIENTED_EDGE('',*,*,#3136,.T.);
#3899=ORIENTED_EDGE('',*,*,#3107,.F.);
#3900=ORIENTED_EDGE('',*,*,#3139,.T.);
#3901=ORIENTED_EDGE('',*,*,#3099,.F.);
#3902=ORIENTED_EDGE('',*,*,#3138,.F.);
#3903=ORIENTED_EDGE('',*,*,#3134,.T.);
#3904=ORIENTED_EDGE('',*,*,#3100,.F.);
#3905=ORIENTED_EDGE('',*,*,#3139,.F.);
#3906=ORIENTED_EDGE('',*,*,#3106,.F.);
#3907=ORIENTED_EDGE('',*,*,#3088,.F.);
#3908=ORIENTED_EDGE('',*,*,#3140,.F.);
#3909=ORIENTED_EDGE('',*,*,#3089,.F.);
#3910=ORIENTED_EDGE('',*,*,#3140,.T.);
#3911=ORIENTED_EDGE('',*,*,#3087,.F.);
#3912=ORIENTED_EDGE('',*,*,#3124,.F.);
#3913=ORIENTED_EDGE('',*,*,#3141,.T.);
#3914=ORIENTED_EDGE('',*,*,#3122,.F.);
#3915=ORIENTED_EDGE('',*,*,#3090,.F.);
#3916=ORIENTED_EDGE('',*,*,#3086,.F.);
#3917=ORIENTED_EDGE('',*,*,#3142,.F.);
#3918=ORIENTED_EDGE('',*,*,#3081,.F.);
#3919=ORIENTED_EDGE('',*,*,#3094,.F.);
#3920=ORIENTED_EDGE('',*,*,#3143,.F.);
#3921=ORIENTED_EDGE('',*,*,#3123,.F.);
#3922=ORIENTED_EDGE('',*,*,#3141,.F.);
#3923=ORIENTED_EDGE('',*,*,#3143,.T.);
#3924=ORIENTED_EDGE('',*,*,#3093,.F.);
#3925=ORIENTED_EDGE('',*,*,#3144,.F.);
#3926=ORIENTED_EDGE('',*,*,#3082,.F.);
#3927=ORIENTED_EDGE('',*,*,#3145,.F.);
#3928=ORIENTED_EDGE('',*,*,#3146,.T.);
#3929=ORIENTED_EDGE('',*,*,#3083,.F.);
#3930=ORIENTED_EDGE('',*,*,#3144,.T.);
#3931=ORIENTED_EDGE('',*,*,#3092,.F.);
#3932=ORIENTED_EDGE('',*,*,#3147,.T.);
#3933=ORIENTED_EDGE('',*,*,#3084,.F.);
#3934=ORIENTED_EDGE('',*,*,#3146,.F.);
#3935=ORIENTED_EDGE('',*,*,#3142,.T.);
#3936=ORIENTED_EDGE('',*,*,#3085,.F.);
#3937=ORIENTED_EDGE('',*,*,#3147,.F.);
#3938=ORIENTED_EDGE('',*,*,#3091,.F.);
#3939=ORIENTED_EDGE('',*,*,#3073,.F.);
#3940=ORIENTED_EDGE('',*,*,#3148,.F.);
#3941=ORIENTED_EDGE('',*,*,#3074,.F.);
#3942=ORIENTED_EDGE('',*,*,#3148,.T.);
#3943=ORIENTED_EDGE('',*,*,#3072,.F.);
#3944=ORIENTED_EDGE('',*,*,#3127,.F.);
#3945=ORIENTED_EDGE('',*,*,#3149,.T.);
#3946=ORIENTED_EDGE('',*,*,#3125,.F.);
#3947=ORIENTED_EDGE('',*,*,#3075,.F.);
#3948=ORIENTED_EDGE('',*,*,#3071,.F.);
#3949=ORIENTED_EDGE('',*,*,#3150,.F.);
#3950=ORIENTED_EDGE('',*,*,#3066,.F.);
#3951=ORIENTED_EDGE('',*,*,#3079,.F.);
#3952=ORIENTED_EDGE('',*,*,#3151,.F.);
#3953=ORIENTED_EDGE('',*,*,#3126,.F.);
#3954=ORIENTED_EDGE('',*,*,#3149,.F.);
#3955=ORIENTED_EDGE('',*,*,#3151,.T.);
#3956=ORIENTED_EDGE('',*,*,#3078,.F.);
#3957=ORIENTED_EDGE('',*,*,#3152,.F.);
#3958=ORIENTED_EDGE('',*,*,#3067,.F.);
#3959=ORIENTED_EDGE('',*,*,#3153,.F.);
#3960=ORIENTED_EDGE('',*,*,#3154,.T.);
#3961=ORIENTED_EDGE('',*,*,#3068,.F.);
#3962=ORIENTED_EDGE('',*,*,#3152,.T.);
#3963=ORIENTED_EDGE('',*,*,#3077,.F.);
#3964=ORIENTED_EDGE('',*,*,#3155,.T.);
#3965=ORIENTED_EDGE('',*,*,#3069,.F.);
#3966=ORIENTED_EDGE('',*,*,#3154,.F.);
#3967=ORIENTED_EDGE('',*,*,#3150,.T.);
#3968=ORIENTED_EDGE('',*,*,#3070,.F.);
#3969=ORIENTED_EDGE('',*,*,#3155,.F.);
#3970=ORIENTED_EDGE('',*,*,#3076,.F.);
#3971=ORIENTED_EDGE('',*,*,#3156,.T.);
#3972=ORIENTED_EDGE('',*,*,#3157,.T.);
#3973=ORIENTED_EDGE('',*,*,#3158,.F.);
#3974=ORIENTED_EDGE('',*,*,#3159,.F.);
#3975=ORIENTED_EDGE('',*,*,#3160,.T.);
#3976=ORIENTED_EDGE('',*,*,#3159,.T.);
#3977=ORIENTED_EDGE('',*,*,#3161,.F.);
#3978=ORIENTED_EDGE('',*,*,#3162,.F.);
#3979=ORIENTED_EDGE('',*,*,#3045,.T.);
#3980=ORIENTED_EDGE('',*,*,#3163,.T.);
#3981=ORIENTED_EDGE('',*,*,#3162,.T.);
#3982=ORIENTED_EDGE('',*,*,#3164,.F.);
#3983=ORIENTED_EDGE('',*,*,#3165,.F.);
#3984=ORIENTED_EDGE('',*,*,#3129,.T.);
#3985=ORIENTED_EDGE('',*,*,#3137,.T.);
#3986=ORIENTED_EDGE('',*,*,#3145,.T.);
#3987=ORIENTED_EDGE('',*,*,#3153,.T.);
#3988=ORIENTED_EDGE('',*,*,#3166,.T.);
#3989=ORIENTED_EDGE('',*,*,#3165,.T.);
#3990=ORIENTED_EDGE('',*,*,#3167,.F.);
#3991=ORIENTED_EDGE('',*,*,#3157,.F.);
#3992=ORIENTED_EDGE('',*,*,#3047,.T.);
#3993=ORIENTED_EDGE('',*,*,#3167,.T.);
#3994=ORIENTED_EDGE('',*,*,#3164,.T.);
#3995=ORIENTED_EDGE('',*,*,#3161,.T.);
#3996=ORIENTED_EDGE('',*,*,#3158,.T.);
#3997=ORIENTED_EDGE('',*,*,#3166,.F.);
#3998=ORIENTED_EDGE('',*,*,#3156,.F.);
#3999=ORIENTED_EDGE('',*,*,#3160,.F.);
#4000=ORIENTED_EDGE('',*,*,#3163,.F.);
#4001=ORIENTED_EDGE('',*,*,#3037,.T.);
#4002=ORIENTED_EDGE('',*,*,#3040,.T.);
#5149=CYLINDRICAL_SURFACE('',#5898,0.25);
#5150=CYLINDRICAL_SURFACE('',#5902,0.25);
#5151=CYLINDRICAL_SURFACE('',#5906,0.93);
#5152=CYLINDRICAL_SURFACE('',#5911,0.93);
#5153=CYLINDRICAL_SURFACE('',#5918,0.789999999999999);
#5154=CYLINDRICAL_SURFACE('',#5921,0.789999999999999);
#5155=CYLINDRICAL_SURFACE('',#5925,0.789999999999999);
#5156=CYLINDRICAL_SURFACE('',#5929,0.789999999999999);
#5157=CYLINDRICAL_SURFACE('',#5934,0.79);
#5158=CYLINDRICAL_SURFACE('',#5961,0.93);
#5159=CYLINDRICAL_SURFACE('',#5967,0.789999999999999);
#5160=CYLINDRICAL_SURFACE('',#5968,0.789999999999999);
#5161=CYLINDRICAL_SURFACE('',#5970,0.789999999999999);
#5162=CYLINDRICAL_SURFACE('',#5972,0.789999999999999);
#5163=CYLINDRICAL_SURFACE('',#5977,0.93);
#5164=CYLINDRICAL_SURFACE('',#5983,0.789999999999999);
#5165=CYLINDRICAL_SURFACE('',#5984,0.789999999999999);
#5166=CYLINDRICAL_SURFACE('',#5986,0.789999999999999);
#5167=CYLINDRICAL_SURFACE('',#5988,0.789999999999999);
#5168=CYLINDRICAL_SURFACE('',#5993,0.93);
#5169=CYLINDRICAL_SURFACE('',#5999,0.79);
#5170=CYLINDRICAL_SURFACE('',#6000,0.79);
#5171=CYLINDRICAL_SURFACE('',#6002,0.79);
#5172=CYLINDRICAL_SURFACE('',#6004,0.79);
#5173=CYLINDRICAL_SURFACE('',#6009,0.93);
#5247=ADVANCED_FACE('',(#747),#5149,.F.);
#5248=ADVANCED_FACE('',(#748),#535,.F.);
#5249=ADVANCED_FACE('',(#749),#5150,.F.);
#5250=ADVANCED_FACE('',(#750),#536,.F.);
#5251=ADVANCED_FACE('',(#751),#5151,.F.);
#5252=ADVANCED_FACE('',(#752,#426),#537,.T.);
#5253=ADVANCED_FACE('',(#753),#5152,.F.);
#5254=ADVANCED_FACE('',(#754,#427),#538,.F.);
#5255=ADVANCED_FACE('',(#755),#539,.F.);
#5256=ADVANCED_FACE('',(#756),#5153,.F.);
#5257=ADVANCED_FACE('',(#757),#5154,.F.);
#5258=ADVANCED_FACE('',(#758),#5155,.F.);
#5259=ADVANCED_FACE('',(#759),#5156,.F.);
#5260=ADVANCED_FACE('',(#760),#540,.F.);
#5261=ADVANCED_FACE('',(#761),#5157,.F.);
#5262=ADVANCED_FACE('',(#762),#541,.F.);
#5263=ADVANCED_FACE('',(#763),#5158,.F.);
#5264=ADVANCED_FACE('',(#764),#542,.F.);
#5265=ADVANCED_FACE('',(#765),#543,.F.);
#5266=ADVANCED_FACE('',(#766),#5159,.F.);
#5267=ADVANCED_FACE('',(#767),#5160,.F.);
#5268=ADVANCED_FACE('',(#768),#5161,.F.);
#5269=ADVANCED_FACE('',(#769),#5162,.F.);
#5270=ADVANCED_FACE('',(#770),#544,.F.);
#5271=ADVANCED_FACE('',(#771),#545,.F.);
#5272=ADVANCED_FACE('',(#772),#5163,.F.);
#5273=ADVANCED_FACE('',(#773),#546,.F.);
#5274=ADVANCED_FACE('',(#774),#547,.F.);
#5275=ADVANCED_FACE('',(#775),#5164,.F.);
#5276=ADVANCED_FACE('',(#776),#5165,.F.);
#5277=ADVANCED_FACE('',(#777),#5166,.F.);
#5278=ADVANCED_FACE('',(#778),#5167,.F.);
#5279=ADVANCED_FACE('',(#779),#548,.F.);
#5280=ADVANCED_FACE('',(#780),#549,.F.);
#5281=ADVANCED_FACE('',(#781),#5168,.F.);
#5282=ADVANCED_FACE('',(#782),#550,.F.);
#5283=ADVANCED_FACE('',(#783),#551,.F.);
#5284=ADVANCED_FACE('',(#784),#5169,.F.);
#5285=ADVANCED_FACE('',(#785),#5170,.F.);
#5286=ADVANCED_FACE('',(#786),#5171,.F.);
#5287=ADVANCED_FACE('',(#787),#5172,.F.);
#5288=ADVANCED_FACE('',(#788),#552,.F.);
#5289=ADVANCED_FACE('',(#789),#553,.F.);
#5290=ADVANCED_FACE('',(#790),#5173,.F.);
#5291=ADVANCED_FACE('',(#791),#554,.F.);
#5292=ADVANCED_FACE('',(#792),#555,.T.);
#5293=ADVANCED_FACE('',(#793,#428),#556,.T.);
#5294=ADVANCED_FACE('',(#794,#429,#430,#431,#432),#557,.T.);
#5295=ADVANCED_FACE('',(#795,#433),#558,.T.);
#5296=ADVANCED_FACE('',(#796),#559,.T.);
#5297=ADVANCED_FACE('',(#797,#434,#435),#560,.F.);
#5579=CLOSED_SHELL('',(#5247,#5248,#5249,#5250,#5251,#5252,#5253,#5254,
#5255,#5256,#5257,#5258,#5259,#5260,#5261,#5262,#5263,#5264,#5265,#5266,
#5267,#5268,#5269,#5270,#5271,#5272,#5273,#5274,#5275,#5276,#5277,#5278,
#5279,#5280,#5281,#5282,#5283,#5284,#5285,#5286,#5287,#5288,#5289,#5290,
#5291,#5292,#5293,#5294,#5295,#5296,#5297));
#5897=AXIS2_PLACEMENT_3D('',#8337,#6573,#6574);
#5898=AXIS2_PLACEMENT_3D('',#8338,#6575,#6576);
#5899=AXIS2_PLACEMENT_3D('',#8340,#6577,#6578);
#5900=AXIS2_PLACEMENT_3D('',#8343,#6580,#6581);
#5901=AXIS2_PLACEMENT_3D('',#8344,#6582,#6583);
#5902=AXIS2_PLACEMENT_3D('',#8345,#6584,#6585);
#5903=AXIS2_PLACEMENT_3D('',#8347,#6586,#6587);
#5904=AXIS2_PLACEMENT_3D('',#8350,#6589,#6590);
#5905=AXIS2_PLACEMENT_3D('',#8351,#6591,#6592);
#5906=AXIS2_PLACEMENT_3D('',#8352,#6593,#6594);
#5907=AXIS2_PLACEMENT_3D('',#8354,#6595,#6596);
#5908=AXIS2_PLACEMENT_3D('',#8357,#6598,#6599);
#5909=AXIS2_PLACEMENT_3D('',#8358,#6600,#6601);
#5910=AXIS2_PLACEMENT_3D('',#8360,#6602,#6603);
#5911=AXIS2_PLACEMENT_3D('',#8361,#6604,#6605);
#5912=AXIS2_PLACEMENT_3D('',#8363,#6606,#6607);
#5913=AXIS2_PLACEMENT_3D('',#8366,#6609,#6610);
#5914=AXIS2_PLACEMENT_3D('',#8367,#6611,#6612);
#5915=AXIS2_PLACEMENT_3D('',#8369,#6613,#6614);
#5916=AXIS2_PLACEMENT_3D('',#8370,#6615,#6616);
#5917=AXIS2_PLACEMENT_3D('',#8374,#6618,#6619);
#5918=AXIS2_PLACEMENT_3D('',#8375,#6620,#6621);
#5919=AXIS2_PLACEMENT_3D('',#8377,#6622,#6623);
#5920=AXIS2_PLACEMENT_3D('',#8378,#6624,#6625);
#5921=AXIS2_PLACEMENT_3D('',#8379,#6626,#6627);
#5922=AXIS2_PLACEMENT_3D('',#8382,#6628,#6629);
#5923=AXIS2_PLACEMENT_3D('',#8384,#6630,#6631);
#5924=AXIS2_PLACEMENT_3D('',#8385,#6632,#6633);
#5925=AXIS2_PLACEMENT_3D('',#8386,#6634,#6635);
#5926=AXIS2_PLACEMENT_3D('',#8388,#6636,#6637);
#5927=AXIS2_PLACEMENT_3D('',#8390,#6638,#6639);
#5928=AXIS2_PLACEMENT_3D('',#8391,#6640,#6641);
#5929=AXIS2_PLACEMENT_3D('',#8392,#6642,#6643);
#5930=AXIS2_PLACEMENT_3D('',#8394,#6644,#6645);
#5931=AXIS2_PLACEMENT_3D('',#8396,#6646,#6647);
#5932=AXIS2_PLACEMENT_3D('',#8397,#6648,#6649);
#5933=AXIS2_PLACEMENT_3D('',#8398,#6650,#6651);
#5934=AXIS2_PLACEMENT_3D('',#8400,#6653,#6654);
#5935=AXIS2_PLACEMENT_3D('',#8404,#6656,#6657);
#5936=AXIS2_PLACEMENT_3D('',#8428,#6660,#6661);
#5937=AXIS2_PLACEMENT_3D('',#8430,#6662,#6663);
#5938=AXIS2_PLACEMENT_3D('',#8433,#6665,#6666);
#5939=AXIS2_PLACEMENT_3D('',#8435,#6667,#6668);
#5940=AXIS2_PLACEMENT_3D('',#8455,#6671,#6672);
#5941=AXIS2_PLACEMENT_3D('',#8459,#6674,#6675);
#5942=AXIS2_PLACEMENT_3D('',#8483,#6678,#6679);
#5943=AXIS2_PLACEMENT_3D('',#8485,#6680,#6681);
#5944=AXIS2_PLACEMENT_3D('',#8488,#6683,#6684);
#5945=AXIS2_PLACEMENT_3D('',#8490,#6685,#6686);
#5946=AXIS2_PLACEMENT_3D('',#8510,#6689,#6690);
#5947=AXIS2_PLACEMENT_3D('',#8514,#6692,#6693);
#5948=AXIS2_PLACEMENT_3D('',#8538,#6696,#6697);
#5949=AXIS2_PLACEMENT_3D('',#8540,#6698,#6699);
#5950=AXIS2_PLACEMENT_3D('',#8543,#6701,#6702);
#5951=AXIS2_PLACEMENT_3D('',#8545,#6703,#6704);
#5952=AXIS2_PLACEMENT_3D('',#8565,#6707,#6708);
#5953=AXIS2_PLACEMENT_3D('',#8608,#6715,#6716);
#5954=AXIS2_PLACEMENT_3D('',#8611,#6718,#6719);
#5955=AXIS2_PLACEMENT_3D('',#8613,#6720,#6721);
#5956=AXIS2_PLACEMENT_3D('',#8616,#6723,#6724);
#5957=AXIS2_PLACEMENT_3D('',#8618,#6725,#6726);
#5958=AXIS2_PLACEMENT_3D('',#8621,#6728,#6729);
#5959=AXIS2_PLACEMENT_3D('',#8622,#6730,#6731);
#5960=AXIS2_PLACEMENT_3D('',#8623,#6732,#6733);
#5961=AXIS2_PLACEMENT_3D('',#8624,#6734,#6735);
#5962=AXIS2_PLACEMENT_3D('',#8626,#6736,#6737);
#5963=AXIS2_PLACEMENT_3D('',#8628,#6739,#6740);
#5964=AXIS2_PLACEMENT_3D('',#8629,#6741,#6742);
#5965=AXIS2_PLACEMENT_3D('',#8630,#6743,#6744);
#5966=AXIS2_PLACEMENT_3D('',#8631,#6745,#6746);
#5967=AXIS2_PLACEMENT_3D('',#8632,#6747,#6748);
#5968=AXIS2_PLACEMENT_3D('',#8633,#6749,#6750);
#5969=AXIS2_PLACEMENT_3D('',#8634,#6751,#6752);
#5970=AXIS2_PLACEMENT_3D('',#8635,#6753,#6754);
#5971=AXIS2_PLACEMENT_3D('',#8636,#6755,#6756);
#5972=AXIS2_PLACEMENT_3D('',#8637,#6757,#6758);
#5973=AXIS2_PLACEMENT_3D('',#8638,#6759,#6760);
#5974=AXIS2_PLACEMENT_3D('',#8639,#6761,#6762);
#5975=AXIS2_PLACEMENT_3D('',#8640,#6763,#6764);
#5976=AXIS2_PLACEMENT_3D('',#8641,#6765,#6766);
#5977=AXIS2_PLACEMENT_3D('',#8642,#6767,#6768);
#5978=AXIS2_PLACEMENT_3D('',#8644,#6769,#6770);
#5979=AXIS2_PLACEMENT_3D('',#8646,#6772,#6773);
#5980=AXIS2_PLACEMENT_3D('',#8647,#6774,#6775);
#5981=AXIS2_PLACEMENT_3D('',#8648,#6776,#6777);
#5982=AXIS2_PLACEMENT_3D('',#8649,#6778,#6779);
#5983=AXIS2_PLACEMENT_3D('',#8650,#6780,#6781);
#5984=AXIS2_PLACEMENT_3D('',#8651,#6782,#6783);
#5985=AXIS2_PLACEMENT_3D('',#8652,#6784,#6785);
#5986=AXIS2_PLACEMENT_3D('',#8653,#6786,#6787);
#5987=AXIS2_PLACEMENT_3D('',#8654,#6788,#6789);
#5988=AXIS2_PLACEMENT_3D('',#8655,#6790,#6791);
#5989=AXIS2_PLACEMENT_3D('',#8656,#6792,#6793);
#5990=AXIS2_PLACEMENT_3D('',#8657,#6794,#6795);
#5991=AXIS2_PLACEMENT_3D('',#8658,#6796,#6797);
#5992=AXIS2_PLACEMENT_3D('',#8659,#6798,#6799);
#5993=AXIS2_PLACEMENT_3D('',#8660,#6800,#6801);
#5994=AXIS2_PLACEMENT_3D('',#8662,#6802,#6803);
#5995=AXIS2_PLACEMENT_3D('',#8664,#6805,#6806);
#5996=AXIS2_PLACEMENT_3D('',#8665,#6807,#6808);
#5997=AXIS2_PLACEMENT_3D('',#8666,#6809,#6810);
#5998=AXIS2_PLACEMENT_3D('',#8667,#6811,#6812);
#5999=AXIS2_PLACEMENT_3D('',#8668,#6813,#6814);
#6000=AXIS2_PLACEMENT_3D('',#8669,#6815,#6816);
#6001=AXIS2_PLACEMENT_3D('',#8670,#6817,#6818);
#6002=AXIS2_PLACEMENT_3D('',#8671,#6819,#6820);
#6003=AXIS2_PLACEMENT_3D('',#8672,#6821,#6822);
#6004=AXIS2_PLACEMENT_3D('',#8673,#6823,#6824);
#6005=AXIS2_PLACEMENT_3D('',#8674,#6825,#6826);
#6006=AXIS2_PLACEMENT_3D('',#8675,#6827,#6828);
#6007=AXIS2_PLACEMENT_3D('',#8676,#6829,#6830);
#6008=AXIS2_PLACEMENT_3D('',#8677,#6831,#6832);
#6009=AXIS2_PLACEMENT_3D('',#8678,#6833,#6834);
#6010=AXIS2_PLACEMENT_3D('',#8680,#6835,#6836);
#6011=AXIS2_PLACEMENT_3D('',#8682,#6838,#6839);
#6012=AXIS2_PLACEMENT_3D('',#8683,#6840,#6841);
#6013=AXIS2_PLACEMENT_3D('',#8684,#6842,#6843);
#6014=AXIS2_PLACEMENT_3D('',#8693,#6848,#6849);
#6015=AXIS2_PLACEMENT_3D('',#8699,#6853,#6854);
#6016=AXIS2_PLACEMENT_3D('',#8705,#6858,#6859);
#6017=AXIS2_PLACEMENT_3D('',#8708,#6862,#6863);
#6018=AXIS2_PLACEMENT_3D('',#8709,#6864,#6865);
#6573=DIRECTION('axis',(0.,0.,1.));
#6574=DIRECTION('refdir',(1.,0.,0.));
#6575=DIRECTION('center_axis',(0.,0.,1.));
#6576=DIRECTION('ref_axis',(1.,0.,0.));
#6577=DIRECTION('center_axis',(0.,0.,1.));
#6578=DIRECTION('ref_axis',(1.,0.,0.));
#6579=DIRECTION('',(0.,0.,1.));
#6580=DIRECTION('center_axis',(0.,0.,1.));
#6581=DIRECTION('ref_axis',(1.,0.,0.));
#6582=DIRECTION('center_axis',(0.,0.,1.));
#6583=DIRECTION('ref_axis',(1.,0.,0.));
#6584=DIRECTION('center_axis',(0.,0.,1.));
#6585=DIRECTION('ref_axis',(1.,0.,0.));
#6586=DIRECTION('center_axis',(0.,0.,1.));
#6587=DIRECTION('ref_axis',(1.,0.,0.));
#6588=DIRECTION('',(0.,0.,1.));
#6589=DIRECTION('center_axis',(0.,0.,1.));
#6590=DIRECTION('ref_axis',(1.,0.,0.));
#6591=DIRECTION('center_axis',(0.,0.,1.));
#6592=DIRECTION('ref_axis',(1.,0.,0.));
#6593=DIRECTION('center_axis',(1.,0.,0.));
#6594=DIRECTION('ref_axis',(0.,0.,-1.));
#6595=DIRECTION('center_axis',(1.,0.,0.));
#6596=DIRECTION('ref_axis',(0.,0.,-1.));
#6597=DIRECTION('',(1.,0.,0.));
#6598=DIRECTION('center_axis',(-1.,0.,0.));
#6599=DIRECTION('ref_axis',(0.,0.,-1.));
#6600=DIRECTION('center_axis',(1.,0.,0.));
#6601=DIRECTION('ref_axis',(0.,0.,-1.));
#6602=DIRECTION('center_axis',(1.,0.,0.));
#6603=DIRECTION('ref_axis',(0.,0.,-1.));
#6604=DIRECTION('center_axis',(1.,0.,0.));
#6605=DIRECTION('ref_axis',(0.,0.,-1.));
#6606=DIRECTION('center_axis',(1.,0.,0.));
#6607=DIRECTION('ref_axis',(0.,0.,-1.));
#6608=DIRECTION('',(1.,0.,0.));
#6609=DIRECTION('center_axis',(1.,0.,0.));
#6610=DIRECTION('ref_axis',(0.,0.,-1.));
#6611=DIRECTION('center_axis',(1.,0.,0.));
#6612=DIRECTION('ref_axis',(0.,0.,-1.));
#6613=DIRECTION('center_axis',(-1.,0.,0.));
#6614=DIRECTION('ref_axis',(0.,0.,-1.));
#6615=DIRECTION('center_axis',(0.,1.,0.));
#6616=DIRECTION('ref_axis',(1.,0.,0.));
#6617=DIRECTION('',(1.,0.,0.));
#6618=DIRECTION('center_axis',(0.,1.,0.));
#6619=DIRECTION('ref_axis',(1.,0.,0.));
#6620=DIRECTION('center_axis',(0.,1.,0.));
#6621=DIRECTION('ref_axis',(1.,0.,0.));
#6622=DIRECTION('center_axis',(-0.707106781186548,0.707106781186548,0.));
#6623=DIRECTION('ref_axis',(0.707106781186547,0.707106781186547,0.));
#6624=DIRECTION('center_axis',(0.707106781186548,0.707106781186547,0.));
#6625=DIRECTION('ref_axis',(0.707106781186547,-0.707106781186548,0.));
#6626=DIRECTION('center_axis',(0.,1.,0.));
#6627=DIRECTION('ref_axis',(1.,0.,0.));
#6628=DIRECTION('center_axis',(0.707106781186548,0.707106781186547,0.));
#6629=DIRECTION('ref_axis',(0.707106781186547,-0.707106781186548,0.));
#6630=DIRECTION('center_axis',(0.,1.,0.));
#6631=DIRECTION('ref_axis',(1.,0.,0.));
#6632=DIRECTION('center_axis',(-0.707106781186548,0.707106781186548,0.));
#6633=DIRECTION('ref_axis',(0.707106781186547,0.707106781186547,0.));
#6634=DIRECTION('center_axis',(0.,1.,0.));
#6635=DIRECTION('ref_axis',(1.,0.,0.));
#6636=DIRECTION('center_axis',(-0.707106781186548,-0.707106781186547,0.));
#6637=DIRECTION('ref_axis',(0.707106781186547,-0.707106781186548,0.));
#6638=DIRECTION('center_axis',(0.707106781186548,-0.707106781186548,0.));
#6639=DIRECTION('ref_axis',(0.707106781186547,0.707106781186547,0.));
#6640=DIRECTION('center_axis',(0.,1.,0.));
#6641=DIRECTION('ref_axis',(1.,0.,0.));
#6642=DIRECTION('center_axis',(0.,1.,0.));
#6643=DIRECTION('ref_axis',(1.,0.,0.));
#6644=DIRECTION('center_axis',(0.707106781186548,-0.707106781186548,0.));
#6645=DIRECTION('ref_axis',(0.707106781186547,0.707106781186547,0.));
#6646=DIRECTION('center_axis',(-0.707106781186548,-0.707106781186547,0.));
#6647=DIRECTION('ref_axis',(0.707106781186547,-0.707106781186548,0.));
#6648=DIRECTION('center_axis',(0.,1.,0.));
#6649=DIRECTION('ref_axis',(1.,0.,0.));
#6650=DIRECTION('center_axis',(0.,1.,0.));
#6651=DIRECTION('ref_axis',(1.,0.,0.));
#6652=DIRECTION('',(-1.,0.,0.));
#6653=DIRECTION('center_axis',(1.,0.,0.));
#6654=DIRECTION('ref_axis',(0.,0.,-1.));
#6655=DIRECTION('',(1.,0.,0.));
#6656=DIRECTION('center_axis',(0.707106781186547,-0.707106781186548,0.));
#6657=DIRECTION('ref_axis',(0.707106781186548,0.707106781186547,0.));
#6658=DIRECTION('',(-1.,0.,0.));
#6659=DIRECTION('',(1.,0.,0.));
#6660=DIRECTION('center_axis',(0.707106781186547,-0.707106781186548,0.));
#6661=DIRECTION('ref_axis',(0.707106781186548,0.707106781186547,0.));
#6662=DIRECTION('center_axis',(0.707106781186548,0.707106781186548,0.));
#6663=DIRECTION('ref_axis',(0.707106781186547,-0.707106781186547,0.));
#6664=DIRECTION('',(1.,0.,0.));
#6665=DIRECTION('center_axis',(-0.707106781186547,0.707106781186548,0.));
#6666=DIRECTION('ref_axis',(0.707106781186548,0.707106781186547,0.));
#6667=DIRECTION('center_axis',(-0.707106781186548,-0.707106781186548,0.));
#6668=DIRECTION('ref_axis',(0.707106781186547,-0.707106781186547,0.));
#6669=DIRECTION('',(1.,0.,0.));
#6670=DIRECTION('',(-1.,0.,0.));
#6671=DIRECTION('center_axis',(-0.707106781186548,-0.707106781186548,0.));
#6672=DIRECTION('ref_axis',(0.707106781186547,-0.707106781186547,0.));
#6673=DIRECTION('',(1.,0.,0.));
#6674=DIRECTION('center_axis',(0.707106781186548,-0.707106781186548,0.));
#6675=DIRECTION('ref_axis',(0.707106781186547,0.707106781186547,0.));
#6676=DIRECTION('',(-1.,0.,0.));
#6677=DIRECTION('',(1.,0.,0.));
#6678=DIRECTION('center_axis',(0.707106781186548,-0.707106781186548,0.));
#6679=DIRECTION('ref_axis',(0.707106781186547,0.707106781186547,0.));
#6680=DIRECTION('center_axis',(0.707106781186548,0.707106781186547,0.));
#6681=DIRECTION('ref_axis',(0.707106781186547,-0.707106781186548,0.));
#6682=DIRECTION('',(1.,0.,0.));
#6683=DIRECTION('center_axis',(-0.707106781186548,0.707106781186548,0.));
#6684=DIRECTION('ref_axis',(0.707106781186547,0.707106781186547,0.));
#6685=DIRECTION('center_axis',(-0.707106781186548,-0.707106781186547,0.));
#6686=DIRECTION('ref_axis',(0.707106781186547,-0.707106781186548,0.));
#6687=DIRECTION('',(1.,0.,0.));
#6688=DIRECTION('',(-1.,0.,0.));
#6689=DIRECTION('center_axis',(-0.707106781186548,-0.707106781186547,0.));
#6690=DIRECTION('ref_axis',(0.707106781186547,-0.707106781186548,0.));
#6691=DIRECTION('',(1.,0.,0.));
#6692=DIRECTION('center_axis',(0.707106781186548,-0.707106781186548,0.));
#6693=DIRECTION('ref_axis',(0.707106781186547,0.707106781186547,0.));
#6694=DIRECTION('',(-1.,0.,0.));
#6695=DIRECTION('',(1.,0.,0.));
#6696=DIRECTION('center_axis',(0.707106781186548,-0.707106781186548,0.));
#6697=DIRECTION('ref_axis',(0.707106781186547,0.707106781186547,0.));
#6698=DIRECTION('center_axis',(0.707106781186548,0.707106781186547,0.));
#6699=DIRECTION('ref_axis',(0.707106781186547,-0.707106781186548,0.));
#6700=DIRECTION('',(1.,0.,0.));
#6701=DIRECTION('center_axis',(-0.707106781186548,0.707106781186548,0.));
#6702=DIRECTION('ref_axis',(0.707106781186547,0.707106781186547,0.));
#6703=DIRECTION('center_axis',(-0.707106781186548,-0.707106781186547,0.));
#6704=DIRECTION('ref_axis',(0.707106781186547,-0.707106781186548,0.));
#6705=DIRECTION('',(1.,0.,0.));
#6706=DIRECTION('',(-1.,0.,0.));
#6707=DIRECTION('center_axis',(-0.707106781186548,-0.707106781186547,0.));
#6708=DIRECTION('ref_axis',(0.707106781186547,-0.707106781186548,0.));
#6709=DIRECTION('',(1.,0.,0.));
#6710=DIRECTION('',(-1.,0.,0.));
#6711=DIRECTION('',(1.,0.,0.));
#6712=DIRECTION('',(1.,0.,0.));
#6713=DIRECTION('',(-1.,0.,0.));
#6714=DIRECTION('',(1.,0.,0.));
#6715=DIRECTION('center_axis',(-0.707106781186548,0.707106781186548,0.));
#6716=DIRECTION('ref_axis',(0.707106781186547,0.707106781186547,0.));
#6717=DIRECTION('',(-1.,0.,0.));
#6718=DIRECTION('center_axis',(0.707106781186548,0.707106781186547,0.));
#6719=DIRECTION('ref_axis',(0.707106781186547,-0.707106781186548,0.));
#6720=DIRECTION('center_axis',(-0.707106781186548,0.707106781186548,0.));
#6721=DIRECTION('ref_axis',(0.707106781186547,0.707106781186547,0.));
#6722=DIRECTION('',(-1.,0.,0.));
#6723=DIRECTION('center_axis',(0.707106781186548,0.707106781186547,0.));
#6724=DIRECTION('ref_axis',(0.707106781186547,-0.707106781186548,0.));
#6725=DIRECTION('center_axis',(-0.707106781186547,0.707106781186548,0.));
#6726=DIRECTION('ref_axis',(0.707106781186548,0.707106781186547,0.));
#6727=DIRECTION('',(-1.,0.,0.));
#6728=DIRECTION('center_axis',(0.707106781186548,0.707106781186548,0.));
#6729=DIRECTION('ref_axis',(0.707106781186547,-0.707106781186547,0.));
#6730=DIRECTION('center_axis',(0.,1.,0.));
#6731=DIRECTION('ref_axis',(1.,0.,0.));
#6732=DIRECTION('center_axis',(0.,1.,0.));
#6733=DIRECTION('ref_axis',(1.,0.,0.));
#6734=DIRECTION('center_axis',(0.,1.,0.));
#6735=DIRECTION('ref_axis',(1.,0.,0.));
#6736=DIRECTION('center_axis',(0.,1.,0.));
#6737=DIRECTION('ref_axis',(1.,0.,0.));
#6738=DIRECTION('',(0.,1.,0.));
#6739=DIRECTION('center_axis',(0.,1.,0.));
#6740=DIRECTION('ref_axis',(1.,0.,0.));
#6741=DIRECTION('center_axis',(0.,1.,0.));
#6742=DIRECTION('ref_axis',(1.,0.,0.));
#6743=DIRECTION('center_axis',(0.,1.,0.));
#6744=DIRECTION('ref_axis',(1.,0.,0.));
#6745=DIRECTION('center_axis',(0.,1.,0.));
#6746=DIRECTION('ref_axis',(1.,0.,0.));
#6747=DIRECTION('center_axis',(0.,1.,0.));
#6748=DIRECTION('ref_axis',(1.,0.,0.));
#6749=DIRECTION('center_axis',(0.,1.,0.));
#6750=DIRECTION('ref_axis',(1.,0.,0.));
#6751=DIRECTION('center_axis',(0.,1.,0.));
#6752=DIRECTION('ref_axis',(1.,0.,0.));
#6753=DIRECTION('center_axis',(0.,1.,0.));
#6754=DIRECTION('ref_axis',(1.,0.,0.));
#6755=DIRECTION('center_axis',(0.,1.,0.));
#6756=DIRECTION('ref_axis',(1.,0.,0.));
#6757=DIRECTION('center_axis',(0.,1.,0.));
#6758=DIRECTION('ref_axis',(1.,0.,0.));
#6759=DIRECTION('center_axis',(0.,1.,0.));
#6760=DIRECTION('ref_axis',(1.,0.,0.));
#6761=DIRECTION('center_axis',(0.,1.,0.));
#6762=DIRECTION('ref_axis',(1.,0.,0.));
#6763=DIRECTION('center_axis',(0.,1.,0.));
#6764=DIRECTION('ref_axis',(1.,0.,0.));
#6765=DIRECTION('center_axis',(0.,1.,0.));
#6766=DIRECTION('ref_axis',(1.,0.,0.));
#6767=DIRECTION('center_axis',(0.,1.,0.));
#6768=DIRECTION('ref_axis',(1.,0.,0.));
#6769=DIRECTION('center_axis',(0.,1.,0.));
#6770=DIRECTION('ref_axis',(1.,0.,0.));
#6771=DIRECTION('',(0.,1.,0.));
#6772=DIRECTION('center_axis',(0.,1.,0.));
#6773=DIRECTION('ref_axis',(1.,0.,0.));
#6774=DIRECTION('center_axis',(0.,1.,0.));
#6775=DIRECTION('ref_axis',(1.,0.,0.));
#6776=DIRECTION('center_axis',(0.,1.,0.));
#6777=DIRECTION('ref_axis',(1.,0.,0.));
#6778=DIRECTION('center_axis',(0.,1.,0.));
#6779=DIRECTION('ref_axis',(1.,0.,0.));
#6780=DIRECTION('center_axis',(0.,1.,0.));
#6781=DIRECTION('ref_axis',(1.,0.,0.));
#6782=DIRECTION('center_axis',(0.,1.,0.));
#6783=DIRECTION('ref_axis',(1.,0.,0.));
#6784=DIRECTION('center_axis',(0.,1.,0.));
#6785=DIRECTION('ref_axis',(1.,0.,0.));
#6786=DIRECTION('center_axis',(0.,1.,0.));
#6787=DIRECTION('ref_axis',(1.,0.,0.));
#6788=DIRECTION('center_axis',(0.,1.,0.));
#6789=DIRECTION('ref_axis',(1.,0.,0.));
#6790=DIRECTION('center_axis',(0.,1.,0.));
#6791=DIRECTION('ref_axis',(1.,0.,0.));
#6792=DIRECTION('center_axis',(0.,1.,0.));
#6793=DIRECTION('ref_axis',(1.,0.,0.));
#6794=DIRECTION('center_axis',(0.,1.,0.));
#6795=DIRECTION('ref_axis',(1.,0.,0.));
#6796=DIRECTION('center_axis',(0.,1.,0.));
#6797=DIRECTION('ref_axis',(1.,0.,0.));
#6798=DIRECTION('center_axis',(0.,1.,0.));
#6799=DIRECTION('ref_axis',(1.,0.,0.));
#6800=DIRECTION('center_axis',(0.,1.,0.));
#6801=DIRECTION('ref_axis',(1.,0.,0.));
#6802=DIRECTION('center_axis',(0.,1.,0.));
#6803=DIRECTION('ref_axis',(1.,0.,0.));
#6804=DIRECTION('',(0.,1.,0.));
#6805=DIRECTION('center_axis',(0.,1.,0.));
#6806=DIRECTION('ref_axis',(1.,0.,0.));
#6807=DIRECTION('center_axis',(0.,1.,0.));
#6808=DIRECTION('ref_axis',(1.,0.,0.));
#6809=DIRECTION('center_axis',(0.,1.,0.));
#6810=DIRECTION('ref_axis',(1.,0.,0.));
#6811=DIRECTION('center_axis',(0.,1.,0.));
#6812=DIRECTION('ref_axis',(1.,0.,0.));
#6813=DIRECTION('center_axis',(0.,1.,0.));
#6814=DIRECTION('ref_axis',(1.,0.,0.));
#6815=DIRECTION('center_axis',(0.,1.,0.));
#6816=DIRECTION('ref_axis',(1.,0.,0.));
#6817=DIRECTION('center_axis',(0.,1.,0.));
#6818=DIRECTION('ref_axis',(1.,0.,0.));
#6819=DIRECTION('center_axis',(0.,1.,0.));
#6820=DIRECTION('ref_axis',(1.,0.,0.));
#6821=DIRECTION('center_axis',(0.,1.,0.));
#6822=DIRECTION('ref_axis',(1.,0.,0.));
#6823=DIRECTION('center_axis',(0.,1.,0.));
#6824=DIRECTION('ref_axis',(1.,0.,0.));
#6825=DIRECTION('center_axis',(0.,1.,0.));
#6826=DIRECTION('ref_axis',(1.,0.,0.));
#6827=DIRECTION('center_axis',(0.,1.,0.));
#6828=DIRECTION('ref_axis',(1.,0.,0.));
#6829=DIRECTION('center_axis',(0.,1.,0.));
#6830=DIRECTION('ref_axis',(1.,0.,0.));
#6831=DIRECTION('center_axis',(0.,1.,0.));
#6832=DIRECTION('ref_axis',(1.,0.,0.));
#6833=DIRECTION('center_axis',(0.,1.,0.));
#6834=DIRECTION('ref_axis',(1.,0.,0.));
#6835=DIRECTION('center_axis',(0.,1.,0.));
#6836=DIRECTION('ref_axis',(1.,0.,0.));
#6837=DIRECTION('',(0.,1.,0.));
#6838=DIRECTION('center_axis',(0.,1.,0.));
#6839=DIRECTION('ref_axis',(1.,0.,0.));
#6840=DIRECTION('center_axis',(0.,1.,0.));
#6841=DIRECTION('ref_axis',(1.,0.,0.));
#6842=DIRECTION('center_axis',(0.,1.,0.));
#6843=DIRECTION('ref_axis',(-1.,0.,0.));
#6844=DIRECTION('',(-1.,0.,0.));
#6845=DIRECTION('',(0.,0.,1.));
#6846=DIRECTION('',(-1.,0.,0.));
#6847=DIRECTION('',(0.,0.,1.));
#6848=DIRECTION('center_axis',(1.,0.,0.));
#6849=DIRECTION('ref_axis',(0.,1.,0.));
#6850=DIRECTION('',(0.,1.,0.));
#6851=DIRECTION('',(0.,1.,0.));
#6852=DIRECTION('',(0.,0.,1.));
#6853=DIRECTION('center_axis',(0.,-1.,0.));
#6854=DIRECTION('ref_axis',(1.,0.,0.));
#6855=DIRECTION('',(1.,0.,0.));
#6856=DIRECTION('',(1.,0.,0.));
#6857=DIRECTION('',(0.,0.,1.));
#6858=DIRECTION('center_axis',(-1.,0.,0.));
#6859=DIRECTION('ref_axis',(0.,-1.,0.));
#6860=DIRECTION('',(0.,-1.,0.));
#6861=DIRECTION('',(0.,-1.,0.));
#6862=DIRECTION('center_axis',(0.,0.,1.));
#6863=DIRECTION('ref_axis',(1.,0.,0.));
#6864=DIRECTION('center_axis',(0.,0.,1.));
#6865=DIRECTION('ref_axis',(1.,0.,0.));
#8337=CARTESIAN_POINT('',(0.,0.,0.));
#8338=CARTESIAN_POINT('Origin',(38.5,9.,3.4));
#8339=CARTESIAN_POINT('',(38.25,9.,3.5));
#8340=CARTESIAN_POINT('Origin',(38.5,9.,3.5));
#8341=CARTESIAN_POINT('',(38.25,9.,5.3));
#8342=CARTESIAN_POINT('',(38.25,9.,3.4));
#8343=CARTESIAN_POINT('Origin',(38.5,9.,5.3));
#8344=CARTESIAN_POINT('Origin',(38.5,9.,5.3));
#8345=CARTESIAN_POINT('Origin',(-2.5,9.,3.4));
#8346=CARTESIAN_POINT('',(-2.75,9.,3.5));
#8347=CARTESIAN_POINT('Origin',(-2.5,9.,3.5));
#8348=CARTESIAN_POINT('',(-2.75,9.,5.3));
#8349=CARTESIAN_POINT('',(-2.75,9.,3.4));
#8350=CARTESIAN_POINT('Origin',(-2.5,9.,5.3));
#8351=CARTESIAN_POINT('Origin',(-2.5,9.,5.3));
#8352=CARTESIAN_POINT('Origin',(38.7,7.75,5.));
#8353=CARTESIAN_POINT('',(38.7,7.75,5.93));
#8354=CARTESIAN_POINT('Origin',(38.7,7.75,5.));
#8355=CARTESIAN_POINT('',(40.,7.75,5.93));
#8356=CARTESIAN_POINT('',(38.7,7.75,5.93));
#8357=CARTESIAN_POINT('Origin',(40.,7.75,5.));
#8358=CARTESIAN_POINT('Origin',(38.7,7.75,5.));
#8359=CARTESIAN_POINT('',(38.7,7.75,5.79));
#8360=CARTESIAN_POINT('Origin',(38.7,7.75,5.));
#8361=CARTESIAN_POINT('Origin',(-4.1,7.75,5.));
#8362=CARTESIAN_POINT('',(-4.,7.75,5.93));
#8363=CARTESIAN_POINT('Origin',(-4.,7.75,5.));
#8364=CARTESIAN_POINT('',(-2.7,7.75,5.93));
#8365=CARTESIAN_POINT('',(-4.1,7.75,5.93));
#8366=CARTESIAN_POINT('Origin',(-2.7,7.75,5.));
#8367=CARTESIAN_POINT('Origin',(-2.7,7.75,5.));
#8368=CARTESIAN_POINT('',(-2.7,7.75,5.79));
#8369=CARTESIAN_POINT('Origin',(-2.7,7.75,5.));
#8370=CARTESIAN_POINT('Origin',(36.,7.9,5.));
#8371=CARTESIAN_POINT('',(35.85,7.9,4.22437122281339));
#8372=CARTESIAN_POINT('',(36.15,7.9,4.22437122281339));
#8373=CARTESIAN_POINT('',(-4.1,7.9,4.22437122281339));
#8374=CARTESIAN_POINT('Origin',(36.,7.9,5.));
#8375=CARTESIAN_POINT('Origin',(36.,7.2,5.));
#8376=CARTESIAN_POINT('',(36.,7.75,4.21));
#8377=CARTESIAN_POINT('Origin',(36.,7.75,5.));
#8378=CARTESIAN_POINT('Origin',(36.,7.75,5.));
#8379=CARTESIAN_POINT('Origin',(36.,7.2,5.));
#8380=CARTESIAN_POINT('',(35.85,7.9,5.77562877718661));
#8381=CARTESIAN_POINT('',(36.,7.75,5.79));
#8382=CARTESIAN_POINT('Origin',(36.,7.75,5.));
#8383=CARTESIAN_POINT('',(36.15,7.9,5.77562877718661));
#8384=CARTESIAN_POINT('Origin',(36.,7.9,5.));
#8385=CARTESIAN_POINT('Origin',(36.,7.75,5.));
#8386=CARTESIAN_POINT('Origin',(36.,7.2,5.));
#8387=CARTESIAN_POINT('',(36.45,7.3,4.35069267677008));
#8388=CARTESIAN_POINT('Origin',(36.,7.75,5.));
#8389=CARTESIAN_POINT('',(35.55,7.3,4.35069267677008));
#8390=CARTESIAN_POINT('Origin',(36.,7.75,5.));
#8391=CARTESIAN_POINT('Origin',(36.,7.3,5.));
#8392=CARTESIAN_POINT('Origin',(36.,7.2,5.));
#8393=CARTESIAN_POINT('',(35.55,7.3,5.64930732322992));
#8394=CARTESIAN_POINT('Origin',(36.,7.75,5.));
#8395=CARTESIAN_POINT('',(36.45,7.3,5.64930732322992));
#8396=CARTESIAN_POINT('Origin',(36.,7.75,5.));
#8397=CARTESIAN_POINT('Origin',(36.,7.3,5.));
#8398=CARTESIAN_POINT('Origin',(36.,7.9,5.));
#8399=CARTESIAN_POINT('',(-4.1,7.9,5.77562877718661));
#8400=CARTESIAN_POINT('Origin',(-4.1,7.75,5.));
#8401=CARTESIAN_POINT('',(0.,7.75,5.79));
#8402=CARTESIAN_POINT('',(-4.1,7.75,5.79));
#8403=CARTESIAN_POINT('',(-0.449999999999999,7.3,5.64930732322992));
#8404=CARTESIAN_POINT('Origin',(0.,7.75,5.));
#8405=CARTESIAN_POINT('',(-0.665807780068691,7.3,5.64930732322992));
#8406=CARTESIAN_POINT('',(-4.1,7.3,5.64930732322992));
#8407=CARTESIAN_POINT('',(-0.93,6.96,5.));
#8408=CARTESIAN_POINT('Ctrl Pts',(-0.665807780068692,7.3,5.64930732322992));
#8409=CARTESIAN_POINT('Ctrl Pts',(-0.692408622377835,7.26064211607598,5.62203048969952));
#8410=CARTESIAN_POINT('Ctrl Pts',(-0.718893727897336,7.22418930146339,5.59141801573814));
#8411=CARTESIAN_POINT('Ctrl Pts',(-0.793043306765111,7.12549314225287,5.49272185652762));
#8412=CARTESIAN_POINT('Ctrl Pts',(-0.842132255743763,7.06521916742952,5.40773913323974));
#8413=CARTESIAN_POINT('Ctrl Pts',(-0.910788192048256,6.98235868447187,5.21424953523639));
#8414=CARTESIAN_POINT('Ctrl Pts',(-0.93,6.96,5.10551936287513));
#8415=CARTESIAN_POINT('Ctrl Pts',(-0.93,6.96,5.));
#8416=CARTESIAN_POINT('',(-0.665807780068691,7.3,4.35069267677008));
#8417=CARTESIAN_POINT('Ctrl Pts',(-0.93,6.96,5.));
#8418=CARTESIAN_POINT('Ctrl Pts',(-0.93,6.96,4.89448063712487));
#8419=CARTESIAN_POINT('Ctrl Pts',(-0.910788192048256,6.98235868447187,4.78575046476361));
#8420=CARTESIAN_POINT('Ctrl Pts',(-0.842132255743762,7.06521916742952,4.59226086676026));
#8421=CARTESIAN_POINT('Ctrl Pts',(-0.793043306765111,7.12549314225287,4.50727814347238));
#8422=CARTESIAN_POINT('Ctrl Pts',(-0.718893727897336,7.22418930146339,4.40858198426186));
#8423=CARTESIAN_POINT('Ctrl Pts',(-0.692408622377835,7.26064211607598,4.37796951030048));
#8424=CARTESIAN_POINT('Ctrl Pts',(-0.665807780068692,7.3,4.35069267677008));
#8425=CARTESIAN_POINT('',(-0.449999999999999,7.3,4.35069267677008));
#8426=CARTESIAN_POINT('',(-4.1,7.3,4.35069267677008));
#8427=CARTESIAN_POINT('',(0.,7.75,4.21));
#8428=CARTESIAN_POINT('Origin',(0.,7.75,5.));
#8429=CARTESIAN_POINT('',(-0.15,7.9,4.22437122281339));
#8430=CARTESIAN_POINT('Origin',(0.,7.75,5.));
#8431=CARTESIAN_POINT('',(0.15,7.9,4.22437122281339));
#8432=CARTESIAN_POINT('',(-4.1,7.9,4.22437122281339));
#8433=CARTESIAN_POINT('Origin',(0.,7.75,5.));
#8434=CARTESIAN_POINT('',(0.449999999999999,7.3,4.35069267677008));
#8435=CARTESIAN_POINT('Origin',(0.,7.75,5.));
#8436=CARTESIAN_POINT('',(0.665807780068691,7.3,4.35069267677008));
#8437=CARTESIAN_POINT('',(-4.1,7.3,4.35069267677008));
#8438=CARTESIAN_POINT('',(0.665807780068691,7.3,5.64930732322992));
#8439=CARTESIAN_POINT('Ctrl Pts',(0.665807780068692,7.3,4.35069267677008));
#8440=CARTESIAN_POINT('Ctrl Pts',(0.692408622377835,7.26064211607598,4.37796951030048));
#8441=CARTESIAN_POINT('Ctrl Pts',(0.718893727897336,7.22418930146339,4.40858198426186));
#8442=CARTESIAN_POINT('Ctrl Pts',(0.793043306765111,7.12549314225287,4.50727814347238));
#8443=CARTESIAN_POINT('Ctrl Pts',(0.842132255743763,7.06521916742952,4.59226086676026));
#8444=CARTESIAN_POINT('Ctrl Pts',(0.910788192048256,6.98235868447187,4.78575046476361));
#8445=CARTESIAN_POINT('Ctrl Pts',(0.93,6.96,4.89448063712487));
#8446=CARTESIAN_POINT('Ctrl Pts',(0.93,6.96,5.10551936287513));
#8447=CARTESIAN_POINT('Ctrl Pts',(0.910788192048256,6.98235868447187,5.21424953523639));
#8448=CARTESIAN_POINT('Ctrl Pts',(0.842132255743762,7.06521916742952,5.40773913323974));
#8449=CARTESIAN_POINT('Ctrl Pts',(0.793043306765111,7.12549314225287,5.49272185652762));
#8450=CARTESIAN_POINT('Ctrl Pts',(0.718893727897336,7.22418930146339,5.59141801573814));
#8451=CARTESIAN_POINT('Ctrl Pts',(0.692408622377835,7.26064211607598,5.62203048969952));
#8452=CARTESIAN_POINT('Ctrl Pts',(0.665807780068692,7.3,5.64930732322992));
#8453=CARTESIAN_POINT('',(0.449999999999999,7.3,5.64930732322992));
#8454=CARTESIAN_POINT('',(-4.1,7.3,5.64930732322992));
#8455=CARTESIAN_POINT('Origin',(0.,7.75,5.));
#8456=CARTESIAN_POINT('',(12.,7.75,5.79));
#8457=CARTESIAN_POINT('',(-4.1,7.75,5.79));
#8458=CARTESIAN_POINT('',(11.55,7.3,5.64930732322992));
#8459=CARTESIAN_POINT('Origin',(12.,7.75,5.));
#8460=CARTESIAN_POINT('',(11.3341922199313,7.3,5.64930732322992));
#8461=CARTESIAN_POINT('',(-4.1,7.3,5.64930732322992));
#8462=CARTESIAN_POINT('',(11.07,6.96,5.));
#8463=CARTESIAN_POINT('Ctrl Pts',(11.3341922199313,7.3,5.64930732322992));
#8464=CARTESIAN_POINT('Ctrl Pts',(11.3075913776222,7.26064211607598,5.62203048969952));
#8465=CARTESIAN_POINT('Ctrl Pts',(11.2811062721027,7.22418930146339,5.59141801573814));
#8466=CARTESIAN_POINT('Ctrl Pts',(11.2069566932349,7.12549314225287,5.49272185652762));
#8467=CARTESIAN_POINT('Ctrl Pts',(11.1578677442562,7.06521916742952,5.40773913323974));
#8468=CARTESIAN_POINT('Ctrl Pts',(11.0892118079517,6.98235868447187,5.21424953523639));
#8469=CARTESIAN_POINT('Ctrl Pts',(11.07,6.96,5.10551936287513));
#8470=CARTESIAN_POINT('Ctrl Pts',(11.07,6.96,5.));
#8471=CARTESIAN_POINT('',(11.3341922199313,7.3,4.35069267677008));
#8472=CARTESIAN_POINT('Ctrl Pts',(11.07,6.96,5.));
#8473=CARTESIAN_POINT('Ctrl Pts',(11.07,6.96,4.89448063712487));
#8474=CARTESIAN_POINT('Ctrl Pts',(11.0892118079517,6.98235868447187,4.78575046476361));
#8475=CARTESIAN_POINT('Ctrl Pts',(11.1578677442562,7.06521916742952,4.59226086676026));
#8476=CARTESIAN_POINT('Ctrl Pts',(11.2069566932349,7.12549314225287,4.50727814347238));
#8477=CARTESIAN_POINT('Ctrl Pts',(11.2811062721027,7.22418930146339,4.40858198426186));
#8478=CARTESIAN_POINT('Ctrl Pts',(11.3075913776222,7.26064211607598,4.37796951030048));
#8479=CARTESIAN_POINT('Ctrl Pts',(11.3341922199313,7.3,4.35069267677008));
#8480=CARTESIAN_POINT('',(11.55,7.3,4.35069267677008));
#8481=CARTESIAN_POINT('',(-4.1,7.3,4.35069267677008));
#8482=CARTESIAN_POINT('',(12.,7.75,4.21));
#8483=CARTESIAN_POINT('Origin',(12.,7.75,5.));
#8484=CARTESIAN_POINT('',(11.85,7.9,4.22437122281339));
#8485=CARTESIAN_POINT('Origin',(12.,7.75,5.));
#8486=CARTESIAN_POINT('',(12.15,7.9,4.22437122281339));
#8487=CARTESIAN_POINT('',(-4.1,7.9,4.22437122281339));
#8488=CARTESIAN_POINT('Origin',(12.,7.75,5.));
#8489=CARTESIAN_POINT('',(12.45,7.3,4.35069267677008));
#8490=CARTESIAN_POINT('Origin',(12.,7.75,5.));
#8491=CARTESIAN_POINT('',(12.6658077800687,7.3,4.35069267677008));
#8492=CARTESIAN_POINT('',(-4.1,7.3,4.35069267677008));
#8493=CARTESIAN_POINT('',(12.6658077800687,7.3,5.64930732322992));
#8494=CARTESIAN_POINT('Ctrl Pts',(12.6658077800687,7.3,4.35069267677008));
#8495=CARTESIAN_POINT('Ctrl Pts',(12.6924086223778,7.26064211607598,4.37796951030047));
#8496=CARTESIAN_POINT('Ctrl Pts',(12.7188937278973,7.22418930146339,4.40858198426186));
#8497=CARTESIAN_POINT('Ctrl Pts',(12.7930433067651,7.12549314225287,4.50727814347238));
#8498=CARTESIAN_POINT('Ctrl Pts',(12.8421322557438,7.06521916742952,4.59226086676026));
#8499=CARTESIAN_POINT('Ctrl Pts',(12.9107881920483,6.98235868447187,4.78575046476361));
#8500=CARTESIAN_POINT('Ctrl Pts',(12.93,6.96,4.89448063712487));
#8501=CARTESIAN_POINT('Ctrl Pts',(12.93,6.96,5.10551936287513));
#8502=CARTESIAN_POINT('Ctrl Pts',(12.9107881920483,6.98235868447187,5.21424953523639));
#8503=CARTESIAN_POINT('Ctrl Pts',(12.8421322557438,7.06521916742952,5.40773913323974));
#8504=CARTESIAN_POINT('Ctrl Pts',(12.7930433067651,7.12549314225287,5.49272185652762));
#8505=CARTESIAN_POINT('Ctrl Pts',(12.7188937278973,7.22418930146339,5.59141801573814));
#8506=CARTESIAN_POINT('Ctrl Pts',(12.6924086223778,7.26064211607599,5.62203048969953));
#8507=CARTESIAN_POINT('Ctrl Pts',(12.6658077800687,7.3,5.64930732322992));
#8508=CARTESIAN_POINT('',(12.45,7.3,5.64930732322992));
#8509=CARTESIAN_POINT('',(-4.1,7.3,5.64930732322992));
#8510=CARTESIAN_POINT('Origin',(12.,7.75,5.));
#8511=CARTESIAN_POINT('',(24.,7.75,5.79));
#8512=CARTESIAN_POINT('',(-4.1,7.75,5.79));
#8513=CARTESIAN_POINT('',(23.55,7.3,5.64930732322992));
#8514=CARTESIAN_POINT('Origin',(24.,7.75,5.));
#8515=CARTESIAN_POINT('',(23.3341922199313,7.3,5.64930732322992));
#8516=CARTESIAN_POINT('',(-4.1,7.3,5.64930732322992));
#8517=CARTESIAN_POINT('',(23.07,6.96,5.));
#8518=CARTESIAN_POINT('Ctrl Pts',(23.3341922199313,7.3,5.64930732322992));
#8519=CARTESIAN_POINT('Ctrl Pts',(23.3075913776222,7.26064211607598,5.62203048969952));
#8520=CARTESIAN_POINT('Ctrl Pts',(23.2811062721027,7.2241893014634,5.59141801573814));
#8521=CARTESIAN_POINT('Ctrl Pts',(23.2069566932349,7.12549314225287,5.49272185652762));
#8522=CARTESIAN_POINT('Ctrl Pts',(23.1578677442562,7.06521916742952,5.40773913323974));
#8523=CARTESIAN_POINT('Ctrl Pts',(23.0892118079517,6.98235868447187,5.21424953523639));
#8524=CARTESIAN_POINT('Ctrl Pts',(23.07,6.96,5.10551936287513));
#8525=CARTESIAN_POINT('Ctrl Pts',(23.07,6.96,5.));
#8526=CARTESIAN_POINT('',(23.3341922199313,7.3,4.35069267677008));
#8527=CARTESIAN_POINT('Ctrl Pts',(23.07,6.96,5.));
#8528=CARTESIAN_POINT('Ctrl Pts',(23.07,6.96,4.89448063712487));
#8529=CARTESIAN_POINT('Ctrl Pts',(23.0892118079517,6.98235868447187,4.78575046476361));
#8530=CARTESIAN_POINT('Ctrl Pts',(23.1578677442562,7.06521916742952,4.59226086676026));
#8531=CARTESIAN_POINT('Ctrl Pts',(23.2069566932349,7.12549314225287,4.50727814347238));
#8532=CARTESIAN_POINT('Ctrl Pts',(23.2811062721027,7.2241893014634,4.40858198426186));
#8533=CARTESIAN_POINT('Ctrl Pts',(23.3075913776222,7.26064211607598,4.37796951030048));
#8534=CARTESIAN_POINT('Ctrl Pts',(23.3341922199313,7.3,4.35069267677008));
#8535=CARTESIAN_POINT('',(23.55,7.3,4.35069267677008));
#8536=CARTESIAN_POINT('',(-4.1,7.3,4.35069267677008));
#8537=CARTESIAN_POINT('',(24.,7.75,4.21));
#8538=CARTESIAN_POINT('Origin',(24.,7.75,5.));
#8539=CARTESIAN_POINT('',(23.85,7.9,4.22437122281339));
#8540=CARTESIAN_POINT('Origin',(24.,7.75,5.));
#8541=CARTESIAN_POINT('',(24.15,7.9,4.22437122281339));
#8542=CARTESIAN_POINT('',(-4.1,7.9,4.22437122281339));
#8543=CARTESIAN_POINT('Origin',(24.,7.75,5.));
#8544=CARTESIAN_POINT('',(24.45,7.3,4.35069267677008));
#8545=CARTESIAN_POINT('Origin',(24.,7.75,5.));
#8546=CARTESIAN_POINT('',(24.6658077800687,7.3,4.35069267677008));
#8547=CARTESIAN_POINT('',(-4.1,7.3,4.35069267677008));
#8548=CARTESIAN_POINT('',(24.6658077800687,7.3,5.64930732322992));
#8549=CARTESIAN_POINT('Ctrl Pts',(24.6658077800687,7.3,4.35069267677008));
#8550=CARTESIAN_POINT('Ctrl Pts',(24.6924086223778,7.26064211607598,4.37796951030048));
#8551=CARTESIAN_POINT('Ctrl Pts',(24.7188937278973,7.22418930146339,4.40858198426186));
#8552=CARTESIAN_POINT('Ctrl Pts',(24.7930433067651,7.12549314225287,4.50727814347238));
#8553=CARTESIAN_POINT('Ctrl Pts',(24.8421322557438,7.06521916742952,4.59226086676026));
#8554=CARTESIAN_POINT('Ctrl Pts',(24.9107881920483,6.98235868447187,4.78575046476361));
#8555=CARTESIAN_POINT('Ctrl Pts',(24.93,6.96,4.89448063712487));
#8556=CARTESIAN_POINT('Ctrl Pts',(24.93,6.96,5.10551936287513));
#8557=CARTESIAN_POINT('Ctrl Pts',(24.9107881920483,6.98235868447187,5.21424953523639));
#8558=CARTESIAN_POINT('Ctrl Pts',(24.8421322557438,7.06521916742952,5.40773913323974));
#8559=CARTESIAN_POINT('Ctrl Pts',(24.7930433067651,7.12549314225287,5.49272185652762));
#8560=CARTESIAN_POINT('Ctrl Pts',(24.7188937278973,7.22418930146339,5.59141801573814));
#8561=CARTESIAN_POINT('Ctrl Pts',(24.6924086223778,7.26064211607598,5.62203048969952));
#8562=CARTESIAN_POINT('Ctrl Pts',(24.6658077800687,7.3,5.64930732322992));
#8563=CARTESIAN_POINT('',(24.45,7.3,5.64930732322992));
#8564=CARTESIAN_POINT('',(-4.1,7.3,5.64930732322992));
#8565=CARTESIAN_POINT('Origin',(24.,7.75,5.));
#8566=CARTESIAN_POINT('',(-4.1,7.75,5.79));
#8567=CARTESIAN_POINT('',(35.3341922199313,7.3,5.64930732322992));
#8568=CARTESIAN_POINT('',(-4.1,7.3,5.64930732322992));
#8569=CARTESIAN_POINT('',(35.07,6.96,5.));
#8570=CARTESIAN_POINT('Ctrl Pts',(35.3341922199313,7.3,5.64930732322992));
#8571=CARTESIAN_POINT('Ctrl Pts',(35.3075913776222,7.26064211607598,5.62203048969952));
#8572=CARTESIAN_POINT('Ctrl Pts',(35.2811062721027,7.2241893014634,5.59141801573814));
#8573=CARTESIAN_POINT('Ctrl Pts',(35.2069566932349,7.12549314225287,5.49272185652762));
#8574=CARTESIAN_POINT('Ctrl Pts',(35.1578677442562,7.06521916742952,5.40773913323974));
#8575=CARTESIAN_POINT('Ctrl Pts',(35.0892118079517,6.98235868447187,5.21424953523639));
#8576=CARTESIAN_POINT('Ctrl Pts',(35.07,6.96,5.10551936287513));
#8577=CARTESIAN_POINT('Ctrl Pts',(35.07,6.96,5.));
#8578=CARTESIAN_POINT('',(35.3341922199313,7.3,4.35069267677008));
#8579=CARTESIAN_POINT('Ctrl Pts',(35.07,6.96,5.));
#8580=CARTESIAN_POINT('Ctrl Pts',(35.07,6.96,4.89448063712487));
#8581=CARTESIAN_POINT('Ctrl Pts',(35.0892118079517,6.98235868447187,4.78575046476361));
#8582=CARTESIAN_POINT('Ctrl Pts',(35.1578677442562,7.06521916742952,4.59226086676026));
#8583=CARTESIAN_POINT('Ctrl Pts',(35.2069566932349,7.12549314225287,4.50727814347238));
#8584=CARTESIAN_POINT('Ctrl Pts',(35.2811062721027,7.22418930146339,4.40858198426186));
#8585=CARTESIAN_POINT('Ctrl Pts',(35.3075913776222,7.26064211607598,4.37796951030048));
#8586=CARTESIAN_POINT('Ctrl Pts',(35.3341922199313,7.3,4.35069267677008));
#8587=CARTESIAN_POINT('',(-4.1,7.3,4.35069267677008));
#8588=CARTESIAN_POINT('',(36.6658077800687,7.3,4.35069267677008));
#8589=CARTESIAN_POINT('',(-4.1,7.3,4.35069267677008));
#8590=CARTESIAN_POINT('',(36.6658077800687,7.3,5.64930732322992));
#8591=CARTESIAN_POINT('Ctrl Pts',(36.6658077800687,7.3,4.35069267677008));
#8592=CARTESIAN_POINT('Ctrl Pts',(36.6924086223778,7.26064211607598,4.37796951030048));
#8593=CARTESIAN_POINT('Ctrl Pts',(36.7188937278973,7.22418930146339,4.40858198426186));
#8594=CARTESIAN_POINT('Ctrl Pts',(36.7930433067651,7.12549314225287,4.50727814347238));
#8595=CARTESIAN_POINT('Ctrl Pts',(36.8421322557438,7.06521916742952,4.59226086676026));
#8596=CARTESIAN_POINT('Ctrl Pts',(36.9107881920483,6.98235868447187,4.78575046476361));
#8597=CARTESIAN_POINT('Ctrl Pts',(36.93,6.96,4.89448063712487));
#8598=CARTESIAN_POINT('Ctrl Pts',(36.93,6.96,5.10551936287513));
#8599=CARTESIAN_POINT('Ctrl Pts',(36.9107881920483,6.98235868447187,5.21424953523639));
#8600=CARTESIAN_POINT('Ctrl Pts',(36.8421322557438,7.06521916742952,5.40773913323974));
#8601=CARTESIAN_POINT('Ctrl Pts',(36.7930433067651,7.12549314225287,5.49272185652762));
#8602=CARTESIAN_POINT('Ctrl Pts',(36.7188937278973,7.22418930146339,5.59141801573814));
#8603=CARTESIAN_POINT('Ctrl Pts',(36.6924086223778,7.26064211607598,5.62203048969952));
#8604=CARTESIAN_POINT('Ctrl Pts',(36.6658077800687,7.3,5.64930732322992));
#8605=CARTESIAN_POINT('',(-4.1,7.3,5.64930732322992));
#8606=CARTESIAN_POINT('',(-4.1,7.75,5.79));
#8607=CARTESIAN_POINT('',(24.15,7.9,5.77562877718661));
#8608=CARTESIAN_POINT('Origin',(24.,7.75,5.));
#8609=CARTESIAN_POINT('',(23.85,7.9,5.77562877718661));
#8610=CARTESIAN_POINT('',(-4.1,7.9,5.77562877718661));
#8611=CARTESIAN_POINT('Origin',(24.,7.75,5.));
#8612=CARTESIAN_POINT('',(12.15,7.9,5.77562877718661));
#8613=CARTESIAN_POINT('Origin',(12.,7.75,5.));
#8614=CARTESIAN_POINT('',(11.85,7.9,5.77562877718661));
#8615=CARTESIAN_POINT('',(-4.1,7.9,5.77562877718661));
#8616=CARTESIAN_POINT('Origin',(12.,7.75,5.));
#8617=CARTESIAN_POINT('',(0.15,7.9,5.77562877718661));
#8618=CARTESIAN_POINT('Origin',(0.,7.75,5.));
#8619=CARTESIAN_POINT('',(-0.15,7.9,5.77562877718661));
#8620=CARTESIAN_POINT('',(-4.1,7.9,5.77562877718661));
#8621=CARTESIAN_POINT('Origin',(0.,7.75,5.));
#8622=CARTESIAN_POINT('Origin',(36.,7.3,5.));
#8623=CARTESIAN_POINT('Origin',(36.,7.3,5.));
#8624=CARTESIAN_POINT('Origin',(36.,5.9,5.));
#8625=CARTESIAN_POINT('',(35.07,6.,5.));
#8626=CARTESIAN_POINT('Origin',(36.,6.,5.));
#8627=CARTESIAN_POINT('',(35.07,5.9,5.));
#8628=CARTESIAN_POINT('Origin',(36.,7.3,5.));
#8629=CARTESIAN_POINT('Origin',(36.,7.3,5.));
#8630=CARTESIAN_POINT('Origin',(24.,7.9,5.));
#8631=CARTESIAN_POINT('Origin',(24.,7.9,5.));
#8632=CARTESIAN_POINT('Origin',(24.,7.2,5.));
#8633=CARTESIAN_POINT('Origin',(24.,7.2,5.));
#8634=CARTESIAN_POINT('Origin',(24.,7.9,5.));
#8635=CARTESIAN_POINT('Origin',(24.,7.2,5.));
#8636=CARTESIAN_POINT('Origin',(24.,7.3,5.));
#8637=CARTESIAN_POINT('Origin',(24.,7.2,5.));
#8638=CARTESIAN_POINT('Origin',(24.,7.3,5.));
#8639=CARTESIAN_POINT('Origin',(24.,7.9,5.));
#8640=CARTESIAN_POINT('Origin',(24.,7.3,5.));
#8641=CARTESIAN_POINT('Origin',(24.,7.3,5.));
#8642=CARTESIAN_POINT('Origin',(24.,5.9,5.));
#8643=CARTESIAN_POINT('',(23.07,6.,5.));
#8644=CARTESIAN_POINT('Origin',(24.,6.,5.));
#8645=CARTESIAN_POINT('',(23.07,5.9,5.));
#8646=CARTESIAN_POINT('Origin',(24.,7.3,5.));
#8647=CARTESIAN_POINT('Origin',(24.,7.3,5.));
#8648=CARTESIAN_POINT('Origin',(12.,7.9,5.));
#8649=CARTESIAN_POINT('Origin',(12.,7.9,5.));
#8650=CARTESIAN_POINT('Origin',(12.,7.2,5.));
#8651=CARTESIAN_POINT('Origin',(12.,7.2,5.));
#8652=CARTESIAN_POINT('Origin',(12.,7.9,5.));
#8653=CARTESIAN_POINT('Origin',(12.,7.2,5.));
#8654=CARTESIAN_POINT('Origin',(12.,7.3,5.));
#8655=CARTESIAN_POINT('Origin',(12.,7.2,5.));
#8656=CARTESIAN_POINT('Origin',(12.,7.3,5.));
#8657=CARTESIAN_POINT('Origin',(12.,7.9,5.));
#8658=CARTESIAN_POINT('Origin',(12.,7.3,5.));
#8659=CARTESIAN_POINT('Origin',(12.,7.3,5.));
#8660=CARTESIAN_POINT('Origin',(12.,5.9,5.));
#8661=CARTESIAN_POINT('',(11.07,6.,5.));
#8662=CARTESIAN_POINT('Origin',(12.,6.,5.));
#8663=CARTESIAN_POINT('',(11.07,5.9,5.));
#8664=CARTESIAN_POINT('Origin',(12.,7.3,5.));
#8665=CARTESIAN_POINT('Origin',(12.,7.3,5.));
#8666=CARTESIAN_POINT('Origin',(0.,7.9,5.));
#8667=CARTESIAN_POINT('Origin',(0.,7.9,5.));
#8668=CARTESIAN_POINT('Origin',(0.,7.2,5.));
#8669=CARTESIAN_POINT('Origin',(0.,7.2,5.));
#8670=CARTESIAN_POINT('Origin',(0.,7.9,5.));
#8671=CARTESIAN_POINT('Origin',(0.,7.2,5.));
#8672=CARTESIAN_POINT('Origin',(0.,7.3,5.));
#8673=CARTESIAN_POINT('Origin',(0.,7.2,5.));
#8674=CARTESIAN_POINT('Origin',(0.,7.3,5.));
#8675=CARTESIAN_POINT('Origin',(0.,7.9,5.));
#8676=CARTESIAN_POINT('Origin',(0.,7.3,5.));
#8677=CARTESIAN_POINT('Origin',(0.,7.3,5.));
#8678=CARTESIAN_POINT('Origin',(0.,5.9,5.));
#8679=CARTESIAN_POINT('',(-0.93,6.,5.));
#8680=CARTESIAN_POINT('Origin',(0.,6.,5.));
#8681=CARTESIAN_POINT('',(-0.93,5.9,5.));
#8682=CARTESIAN_POINT('Origin',(0.,7.3,5.));
#8683=CARTESIAN_POINT('Origin',(0.,7.3,5.));
#8684=CARTESIAN_POINT('Origin',(40.,9.5,3.5));
#8685=CARTESIAN_POINT('',(40.,9.5,3.5));
#8686=CARTESIAN_POINT('',(-4.,9.5,3.5));
#8687=CARTESIAN_POINT('',(40.,9.5,3.5));
#8688=CARTESIAN_POINT('',(-4.,9.5,6.5));
#8689=CARTESIAN_POINT('',(-4.,9.5,3.5));
#8690=CARTESIAN_POINT('',(40.,9.5,6.5));
#8691=CARTESIAN_POINT('',(40.,9.5,6.5));
#8692=CARTESIAN_POINT('',(40.,9.5,3.5));
#8693=CARTESIAN_POINT('Origin',(40.,6.,3.5));
#8694=CARTESIAN_POINT('',(40.,6.,3.5));
#8695=CARTESIAN_POINT('',(40.,6.,3.5));
#8696=CARTESIAN_POINT('',(40.,6.,6.5));
#8697=CARTESIAN_POINT('',(40.,6.,6.5));
#8698=CARTESIAN_POINT('',(40.,6.,3.5));
#8699=CARTESIAN_POINT('Origin',(-4.,6.,3.5));
#8700=CARTESIAN_POINT('',(-4.,6.,3.5));
#8701=CARTESIAN_POINT('',(-4.,6.,3.5));
#8702=CARTESIAN_POINT('',(-4.,6.,6.5));
#8703=CARTESIAN_POINT('',(-4.,6.,6.5));
#8704=CARTESIAN_POINT('',(-4.,6.,3.5));
#8705=CARTESIAN_POINT('Origin',(-4.,9.5,3.5));
#8706=CARTESIAN_POINT('',(-4.,9.5,3.5));
#8707=CARTESIAN_POINT('',(-4.,9.5,6.5));
#8708=CARTESIAN_POINT('Origin',(18.,7.75,6.5));
#8709=CARTESIAN_POINT('Origin',(18.,7.75,3.5));
#10060=UNCERTAINTY_MEASURE_WITH_UNIT(LENGTH_MEASURE(0.001),#10120,
'DISTANCE_ACCURACY_VALUE',
'Maximum model space distance between geometric entities at asserted c
onnectivities');
#10088=UNCERTAINTY_MEASURE_WITH_UNIT(LENGTH_MEASURE(0.001),#10120,
'DISTANCE_ACCURACY_VALUE',
'Maximum model space distance between geometric entities at asserted c
onnectivities');
#10091=(
GEOMETRIC_REPRESENTATION_CONTEXT(3)
GLOBAL_UNCERTAINTY_ASSIGNED_CONTEXT((#10060))
GLOBAL_UNIT_ASSIGNED_CONTEXT((#10120,#10122,#10123))
REPRESENTATION_CONTEXT('','3D')
);
#10119=(
GEOMETRIC_REPRESENTATION_CONTEXT(3)
GLOBAL_UNCERTAINTY_ASSIGNED_CONTEXT((#10088))
GLOBAL_UNIT_ASSIGNED_CONTEXT((#10120,#10122,#10123))
REPRESENTATION_CONTEXT('','3D')
);
#10120=(
LENGTH_UNIT()
NAMED_UNIT(*)
SI_UNIT(.CENTI.,.METRE.)
);
#10122=(
NAMED_UNIT(*)
PLANE_ANGLE_UNIT()
SI_UNIT($,.RADIAN.)
);
#10123=(
NAMED_UNIT(*)
SI_UNIT($,.STERADIAN.)
SOLID_ANGLE_UNIT()
);
#10126=SHAPE_DEFINITION_REPRESENTATION(#10156,#10242);
#10156=PRODUCT_DEFINITION_SHAPE('',$,#10273);
#10242=SHAPE_REPRESENTATION('',(#5897),#10091);
#10270=PRODUCT_DEFINITION_CONTEXT('part definition',#10362,'design');
#10273=PRODUCT_DEFINITION('Four-port header','Four-port header',#10303,
#10270);
#10303=PRODUCT_DEFINITION_FORMATION('',$,#10366);
#10362=APPLICATION_CONTEXT(
'Core Data for Automotive Mechanical Design Process');
#10363=PRODUCT_CONTEXT('part definition',#10362,'mechanical');
#10366=PRODUCT('Four-port header','Four-port header','Four-port header',
(#10363));
#10478=COLOUR_RGB('Off White',0.89,0.88,0.83);
#10479=FILL_AREA_STYLE_COLOUR('',#10478);
#10480=FILL_AREA_STYLE('',(#10479));
#10481=SURFACE_STYLE_FILL_AREA(#10480);
#10482=SURFACE_SIDE_STYLE('',(#10481));
#10483=SURFACE_STYLE_USAGE(.BOTH.,#10482);
#10484=PRESENTATION_STYLE_ASSIGNMENT((#10483));
ENDSEC;
END-ISO-10303-21;
